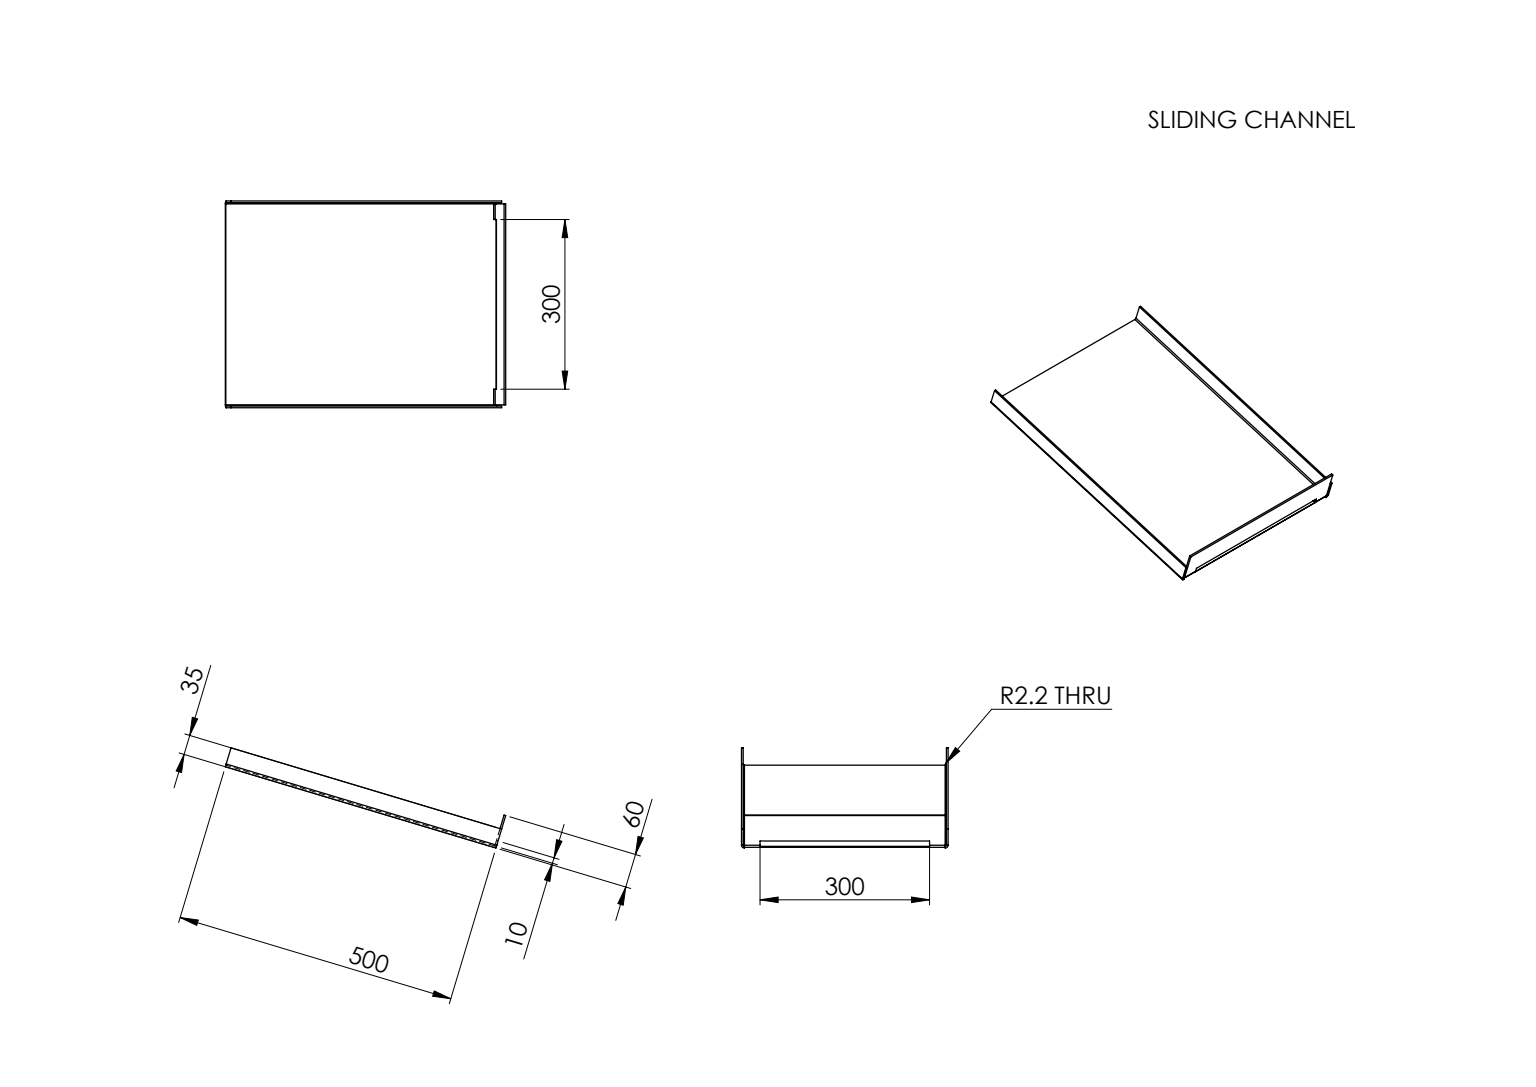
ISO-10303-21;
HEADER;
FILE_DESCRIPTION (('STEP AP214'),
    '1' );
FILE_NAME ('sliding channel.step',
    '2026-10-27T17:01:19',
    ( '' ),
    ( '' ),
    'SwSTEP 2.0',
    'SolidWorks 2026',
    '' );
FILE_SCHEMA (( 'AUTOMOTIVE_DESIGN' ));
ENDSEC;

DATA;
#28=( NAMED_UNIT ( * ) SI_UNIT ( $, .STERADIAN. ) SOLID_ANGLE_UNIT ( ) );
#45=CARTESIAN_POINT ( 'NONE',  ( 702.5260191523640287, 164.1854586329053518, -177.6000000000005059 ) ) ;
#91=ORIENTED_EDGE ( 'NONE', *, *, #14281, .F. ) ;
#93=DIRECTION ( 'NONE',  ( 0.9578262852211525402, -0.2873478855663419429, -0.000000000000000000 ) ) ;
#109=DIRECTION ( 'NONE',  ( 0.000000000000000000, 0.000000000000000000, 1.000000000000000000 ) ) ;
#110=EDGE_LOOP ( 'NONE', ( #11251, #9027, #7663, #8176 ) ) ;
#120=DIRECTION ( 'NONE',  ( -1.673149720584257832E-16, 4.625616335171366110E-15, 1.000000000000000000 ) ) ;
#125=CARTESIAN_POINT ( 'NONE',  ( 716.7018481736364492, 193.3416907550361827, -179.8000000000001535 ) ) ;
#139=LINE ( 'NONE', #7921, #12453 ) ;
#149=DIRECTION ( 'NONE',  ( 0.000000000000000000, 1.000000000000000000, -4.159212477520619976E-15 ) ) ;
#161=CARTESIAN_POINT ( 'NONE',  ( 112.3905262037967248, 374.6350873459896320, 182.7999999999994714 ) ) ;
#166=FACE_OUTER_BOUND ( 'NONE', #2918, .T. ) ;
#167=AXIS2_PLACEMENT_3D ( 'NONE', #3930, #8417, #10718 ) ;
#172=DIRECTION ( 'NONE',  ( 3.340694023494469140E-16, -4.069768234201303760E-15, -1.000000000000000000 ) ) ;
#175=LINE ( 'NONE', #4721, #7503 ) ;
#188=VECTOR ( 'NONE', #2606, 1000.000000000000000 ) ;
#196=ORIENTED_EDGE ( 'NONE', *, *, #8935, .F. ) ;
#199=CARTESIAN_POINT ( 'NONE',  ( 726.1975094929949819, 167.5243180396262801, -149.9999999999986358 ) ) ;
#226=ORIENTED_EDGE ( 'NONE', *, *, #14281, .T. ) ;
#256=VECTOR ( 'NONE', #3741, 1000.000000000000000 ) ;
#288=DIRECTION ( 'NONE',  ( -0.2873478855663281206, -0.9578262852211566480, -1.261617073437843370E-13 ) ) ;
#298=ORIENTED_EDGE ( 'NONE', *, *, #11153, .T. ) ;
#310=CARTESIAN_POINT ( 'NONE',  ( 229.2257385731833779, 308.4724102386176128, -177.6000000000002217 ) ) ;
#334=DIRECTION ( 'NONE',  ( 1.501925087425806625E-16, 4.055197736049677764E-15, 1.000000000000000000 ) ) ;
#367=DIRECTION ( 'NONE',  ( -1.102263794767363534E-15, -3.674212649225433764E-15, -1.000000000000000000 ) ) ;
#376=ORIENTED_EDGE ( 'NONE', *, *, #2427, .F. ) ;
#380=AXIS2_PLACEMENT_3D ( 'NONE', #4209, #11878, #1767 ) ;
#381=DIRECTION ( 'NONE',  ( -0.9578262852211513190, 0.2873478855663454956, -1.110223024625156540E-15 ) ) ;
#394=DIRECTION ( 'NONE',  ( -0.9578262852211506528, 0.2873478855663477161, -0.000000000000000000 ) ) ;
#425=DIRECTION ( 'NONE',  ( -0.9578262852211525402, 0.2873478855663419429, 0.000000000000000000 ) ) ;
#430=EDGE_CURVE ( 'NONE', #7561, #12673, #10485, .T. ) ;
#455=CIRCLE ( 'NONE', #2828, 2.199999999999757705 ) ;
#461=ORIENTED_EDGE ( 'NONE', *, *, #7179, .T. ) ;
#527=CARTESIAN_POINT ( 'NONE',  ( 710.3801946911773939, 172.2695124801716702, -149.9999999999992610 ) ) ;
#547=EDGE_CURVE ( 'NONE', #6337, #5936, #10420, .T. ) ;
#554=DIRECTION ( 'NONE',  ( 0.2873478855663502141, 0.9578262852211498757, -8.036520471939056366E-30 ) ) ;
#567=PLANE ( 'NONE',  #5021 ) ;
#582=CARTESIAN_POINT ( 'NONE',  ( 228.5935732249375292, 306.3651924111313178, -177.6000000000005059 ) ) ;
#597=CARTESIAN_POINT ( 'NONE',  ( 227.7315295682386704, 303.4917135554700280, 177.6000000000001648 ) ) ;
#618=( NAMED_UNIT ( * ) PLANE_ANGLE_UNIT ( ) SI_UNIT ( $, .RADIAN. ) );
#639=ORIENTED_EDGE ( 'NONE', *, *, #9821, .F. ) ;
#647=EDGE_CURVE ( 'NONE', #9997, #6920, #13349, .T. ) ;
#666=EDGE_LOOP ( 'NONE', ( #7423, #9314, #1783, #13496 ) ) ;
#673=CARTESIAN_POINT ( 'NONE',  ( 723.8855453127954434, 217.2873478855664473, 177.5999999999999659 ) ) ;
#683=EDGE_CURVE ( 'NONE', #8002, #5236, #4892, .T. ) ;
#698=EDGE_CURVE ( 'NONE', #10093, #9718, #13285, .T. ) ;
#702=ORIENTED_EDGE ( 'NONE', *, *, #13069, .F. ) ;
#711=EDGE_LOOP ( 'NONE', ( #2678, #10963, #7797, #8249 ) ) ;
#715=VECTOR ( 'NONE', #5972, 1000.000000000000000 ) ;
#733=DIRECTION ( 'NONE',  ( -0.9578262852211513190, 0.2873478855663453846, -1.110223024625157329E-15 ) ) ;
#754=ORIENTED_EDGE ( 'NONE', *, *, #8240, .F. ) ;
#764=EDGE_CURVE ( 'NONE', #11071, #8976, #2432, .T. ) ;
#769=EDGE_CURVE ( 'NONE', #10293, #10481, #1167, .T. ) ;
#777=EDGE_LOOP ( 'NONE', ( #999, #2194, #1865, #13253 ) ) ;
#794=CARTESIAN_POINT ( 'NONE',  ( 237.7887055630607733, 337.0156335382104089, 182.7999999999996135 ) ) ;
#795=CARTESIAN_POINT ( 'NONE',  ( 229.2257385731836621, 308.4724102386199434, 182.7999999999996135 ) ) ;
#826=ORIENTED_EDGE ( 'NONE', *, *, #3158, .T. ) ;
#831=ORIENTED_EDGE ( 'NONE', *, *, #4383, .F. ) ;
#834=DIRECTION ( 'NONE',  ( -0.9578262852211507639, 0.2873478855663477716, 0.000000000000000000 ) ) ;
#837=ORIENTED_EDGE ( 'NONE', *, *, #10575, .F. ) ;
#880=EDGE_CURVE ( 'NONE', #1859, #4991, #1474, .T. ) ;
#884=ORIENTED_EDGE ( 'NONE', *, *, #11917, .F. ) ;
#897=AXIS2_PLACEMENT_3D ( 'NONE', #6006, #10504, #7188 ) ;
#898=VECTOR ( 'NONE', #9160, 1000.000000000000114 ) ;
#899=LINE ( 'NONE', #11699, #906 ) ;
#906=VECTOR ( 'NONE', #6251, 1000.000000000000227 ) ;
#944=AXIS2_PLACEMENT_3D ( 'NONE', #11376, #3638, #8117 ) ;
#971=PLANE ( 'NONE',  #3973 ) ;
#999=ORIENTED_EDGE ( 'NONE', *, *, #2229, .F. ) ;
#1013=ORIENTED_EDGE ( 'NONE', *, *, #8894, .F. ) ;
#1016=FACE_OUTER_BOUND ( 'NONE', #7060, .T. ) ;
#1061=ADVANCED_BREP_SHAPE_REPRESENTATION ( '', ( #7422, #9440 ), #13701 ) ;
#1096=EDGE_LOOP ( 'NONE', ( #2757, #837, #2555, #2386, #1528, #4159 ) ) ;
#1140=DIRECTION ( 'NONE',  ( 0.9578262852211485434, -0.2873478855663546550, 0.000000000000000000 ) ) ;
#1150=AXIS2_PLACEMENT_3D ( 'NONE', #673, #6229, #6519 ) ;
#1157=ORIENTED_EDGE ( 'NONE', *, *, #5120, .F. ) ;
#1167=LINE ( 'NONE', #4581, #5578 ) ;
#1172=ORIENTED_EDGE ( 'NONE', *, *, #4383, .T. ) ;
#1174=VECTOR ( 'NONE', #12504, 1000.000000000000114 ) ;
#1197=DIRECTION ( 'NONE',  ( 0.000000000000000000, 0.000000000000000000, 1.000000000000000000 ) ) ;
#1217=EDGE_LOOP ( 'NONE', ( #14260, #12001, #10390, #9108 ) ) ;
#1237=DIRECTION ( 'NONE',  ( 0.9578262852211507639, -0.2873478855663477716, 0.000000000000000000 ) ) ;
#1239=DIRECTION ( 'NONE',  ( -3.340694023494469140E-16, 4.069768234201303760E-15, 1.000000000000000000 ) ) ;
#1255=ORIENTED_EDGE ( 'NONE', *, *, #4794, .T. ) ;
#1292=ORIENTED_EDGE ( 'NONE', *, *, #7379, .F. ) ;
#1303=( LENGTH_UNIT ( ) NAMED_UNIT ( * ) SI_UNIT ( .MILLI., .METRE. ) );
#1316=DIRECTION ( 'NONE',  ( 9.304756960132325412E-16, 6.965275210156238168E-15, 1.000000000000000000 ) ) ;
#1329=DIRECTION ( 'NONE',  ( 0.000000000000000000, -1.000000000000000000, 4.625616335171366110E-15 ) ) ;
#1331=FACE_OUTER_BOUND ( 'NONE', #711, .T. ) ;
#1355=ORIENTED_EDGE ( 'NONE', *, *, #8452, .F. ) ;
#1370=( NAMED_UNIT ( * ) PLANE_ANGLE_UNIT ( ) SI_UNIT ( $, .RADIAN. ) );
#1452=DIRECTION ( 'NONE',  ( -0.2873478855663461062, -0.9578262852211510969, 0.000000000000000000 ) ) ;
#1454=CARTESIAN_POINT ( 'NONE',  ( 229.2257385731836621, 308.4724102386185223, -182.8000000000004945 ) ) ;
#1457=EDGE_CURVE ( 'NONE', #9718, #6337, #5337, .T. ) ;
#1462=ADVANCED_FACE ( 'NONE', ( #13237 ), #971, .F. ) ;
#1470=CARTESIAN_POINT ( 'NONE',  ( 706.6446721788142895, 159.8177707722969672, 177.6000000000001933 ) ) ;
#1474=LINE ( 'NONE', #3622, #8347 ) ;
#1475=EDGE_LOOP ( 'NONE', ( #7036, #7021, #298, #13292 ) ) ;
#1479=ORIENTED_EDGE ( 'NONE', *, *, #764, .F. ) ;
#1482=ORIENTED_EDGE ( 'NONE', *, *, #8935, .T. ) ;
#1515=EDGE_CURVE ( 'NONE', #12673, #2108, #9837, .T. ) ;
#1525=EDGE_CURVE ( 'NONE', #2008, #2622, #11004, .T. ) ;
#1528=ORIENTED_EDGE ( 'NONE', *, *, #4356, .F. ) ;
#1535=CARTESIAN_POINT ( 'NONE',  ( 726.1975094929949819, 167.5243180396262801, -149.9999999999986358 ) ) ;
#1558=DIRECTION ( 'NONE',  ( 0.000000000000000000, 0.000000000000000000, 1.000000000000000000 ) ) ;
#1577=EDGE_CURVE ( 'NONE', #12373, #10093, #9834, .T. ) ;
#1582=EDGE_CURVE ( 'NONE', #14148, #11328, #2371, .T. ) ;
#1598=ADVANCED_FACE ( 'NONE', ( #13528 ), #2447, .F. ) ;
#1607=ORIENTED_EDGE ( 'NONE', *, *, #3104, .F. ) ;
#1608=LINE ( 'NONE', #6260, #8458 ) ;
#1614=AXIS2_PLACEMENT_3D ( 'NONE', #5274, #13367, #12115 ) ;
#1640=VECTOR ( 'NONE', #9507, 1000.000000000000114 ) ;
#1652=VERTEX_POINT ( 'NONE', #3566 ) ;
#1654=ORIENTED_EDGE ( 'NONE', *, *, #6129, .F. ) ;
#1661=CARTESIAN_POINT ( 'NONE',  ( 604.3113219698392413, -181.2933965909535914, -182.7999999999974250 ) ) ;
#1680=DIRECTION ( 'NONE',  ( -1.000000000000000000, 5.337610695313498298E-15, 0.000000000000000000 ) ) ;
#1687=ADVANCED_FACE ( 'NONE', ( #6948 ), #5621, .T. ) ;
#1725=DIRECTION ( 'NONE',  ( -0.2873478855663455511, -0.9578262852211514300, 4.074758502541097232E-16 ) ) ;
#1744=CARTESIAN_POINT ( 'NONE',  ( 706.6446721788141758, 159.8177707722969956, 177.6000000000005627 ) ) ;
#1766=UNCERTAINTY_MEASURE_WITH_UNIT (LENGTH_MEASURE( 1.000000000000000082E-05 ), #1303, 'distance_accuracy_value', 'NONE');
#1767=DIRECTION ( 'NONE',  ( -1.000000000000000000, 0.000000000000000000, 0.000000000000000000 ) ) ;
#1783=ORIENTED_EDGE ( 'NONE', *, *, #10703, .F. ) ;
#1811=VECTOR ( 'NONE', #8380, 1000.000000000000227 ) ;
#1821=EDGE_CURVE ( 'NONE', #12673, #7913, #13600, .T. ) ;
#1844=CARTESIAN_POINT ( 'NONE',  ( 604.3113219698374223, -181.2933965909537903, 177.6000000000015575 ) ) ;
#1851=CIRCLE ( 'NONE', #7037, 5.199999999999760369 ) ;
#1859=VERTEX_POINT ( 'NONE', #1923 ) ;
#1860=AXIS2_PLACEMENT_3D ( 'NONE', #10254, #5816, #9141 ) ;
#1862=CARTESIAN_POINT ( 'NONE',  ( 721.0120664571321640, 218.1493915422654766, 177.5999999999999659 ) ) ;
#1865=ORIENTED_EDGE ( 'NONE', *, *, #6557, .T. ) ;
#1883=PLANE ( 'NONE',  #4671 ) ;
#1891=DIRECTION ( 'NONE',  ( -0.9578262852211513190, 0.2873478855663453846, 0.000000000000000000 ) ) ;
#1923=CARTESIAN_POINT ( 'NONE',  ( 716.7018481736365629, 193.3416907550376322, 182.8000000000001535 ) ) ;
#1951=VECTOR ( 'NONE', #3608, 1000.000000000000227 ) ;
#1955=EDGE_LOOP ( 'NONE', ( #9013, #4556, #6062, #1255 ) ) ;
#1957=CARTESIAN_POINT ( 'NONE',  ( 702.5260191523640287, 164.1854586329053518, -177.6000000000005059 ) ) ;
#1995=VERTEX_POINT ( 'NONE', #6715 ) ;
#2008=VERTEX_POINT ( 'NONE', #4585 ) ;
#2029=DIRECTION ( 'NONE',  ( 0.9578262852211513190, -0.2873478855663453846, 1.110223024625157329E-15 ) ) ;
#2031=ORIENTED_EDGE ( 'NONE', *, *, #1457, .T. ) ;
#2082=ORIENTED_EDGE ( 'NONE', *, *, #12974, .F. ) ;
#2097=AXIS2_PLACEMENT_3D ( 'NONE', #9208, #1237, #3527 ) ;
#2108=VERTEX_POINT ( 'NONE', #6933 ) ;
#2137=ORIENTED_EDGE ( 'NONE', *, *, #7550, .F. ) ;
#2190=DIRECTION ( 'NONE',  ( 0.2873478855663497700, 0.9578262852211499867, 5.078292077360263497E-30 ) ) ;
#2191=FILL_AREA_STYLE_COLOUR ( '', #11800 ) ;
#2194=ORIENTED_EDGE ( 'NONE', *, *, #12145, .F. ) ;
#2200=CARTESIAN_POINT ( 'NONE',  ( 604.3113219698376497, -181.2933965909545861, -149.9999999999986642 ) ) ;
#2202=DIRECTION ( 'NONE',  ( -1.000000000000000000, 0.000000000000000000, 0.000000000000000000 ) ) ;
#2204=ORIENTED_EDGE ( 'NONE', *, *, #7111, .F. ) ;
#2206=PLANE ( 'NONE',  #6110 ) ;
#2211=CARTESIAN_POINT ( 'NONE',  ( 237.7887055630606028, 337.0156335382089310, -179.8000000000007219 ) ) ;
#2229=EDGE_CURVE ( 'NONE', #10293, #1652, #14305, .T. ) ;
#2253=LINE ( 'NONE', #13712, #1951 ) ;
#2258=CARTESIAN_POINT ( 'NONE',  ( 237.7887055630605460, 337.0156335382089310, -179.8000000000007219 ) ) ;
#2295=DIRECTION ( 'NONE',  ( 1.501925087425806625E-16, 4.055197736049677764E-15, 1.000000000000000000 ) ) ;
#2311=CARTESIAN_POINT ( 'NONE',  ( 703.1581845006096501, 166.2926764603917036, -177.6000000000005059 ) ) ;
#2312=AXIS2_PLACEMENT_3D ( 'NONE', #7015, #12474, #288 ) ;
#2371=LINE ( 'NONE', #11516, #898 ) ;
#2379=CARTESIAN_POINT ( 'NONE',  ( 701.6639754956653405, 161.3119797772417883, -177.6000000000005059 ) ) ;
#2386=ORIENTED_EDGE ( 'NONE', *, *, #7087, .T. ) ;
#2423=CARTESIAN_POINT ( 'NONE',  ( 703.1581845006096501, 166.2926764603917036, 150.0000000000013927 ) ) ;
#2427=EDGE_CURVE ( 'NONE', #7561, #9391, #14094, .T. ) ;
#2430=CARTESIAN_POINT ( 'NONE',  ( -1.716263591756835415E-13, -1.266779246227765552E-12, -179.7999999999981355 ) ) ;
#2432=LINE ( 'NONE', #45, #11930 ) ;
#2447=PLANE ( 'NONE',  #10533 ) ;
#2452=VERTEX_POINT ( 'NONE', #12928 ) ;
#2456=CARTESIAN_POINT ( 'NONE',  ( 228.5935732249376429, 306.3651924111320000, -184.8000000000004945 ) ) ;
#2484=DIRECTION ( 'NONE',  ( 1.000000000000000000, 0.000000000000000000, 0.000000000000000000 ) ) ;
#2485=DIRECTION ( 'NONE',  ( 0.9578262852211524292, -0.2873478855663418874, -0.000000000000000000 ) ) ;
#2490=PLANE ( 'NONE',  #13493 ) ;
#2515=ORIENTED_EDGE ( 'NONE', *, *, #3104, .T. ) ;
#2534=ORIENTED_EDGE ( 'NONE', *, *, #13069, .T. ) ;
#2553=VERTEX_POINT ( 'NONE', #6657 ) ;
#2555=ORIENTED_EDGE ( 'NONE', *, *, #9808, .T. ) ;
#2569=FACE_OUTER_BOUND ( 'NONE', #9843, .T. ) ;
#2585=AXIS2_PLACEMENT_3D ( 'NONE', #2423, #4865, #3453 ) ;
#2599=VECTOR ( 'NONE', #7198, 1000.000000000000114 ) ;
#2602=ORIENTED_EDGE ( 'NONE', *, *, #430, .T. ) ;
#2605=CARTESIAN_POINT ( 'NONE',  ( 723.8855453127955570, 217.2873478855649694, -177.6000000000007901 ) ) ;
#2606=DIRECTION ( 'NONE',  ( -0.9578262852210943645, 0.2873478855665353993, 0.000000000000000000 ) ) ;
#2620=CYLINDRICAL_SURFACE ( 'NONE', #897, 2.199999999999701306 ) ;
#2622=VERTEX_POINT ( 'NONE', #4882 ) ;
#2633=LINE ( 'NONE', #6014, #14313 ) ;
#2678=ORIENTED_EDGE ( 'NONE', *, *, #5120, .T. ) ;
#2681=ADVANCED_FACE ( 'NONE', ( #7519 ), #9671, .F. ) ;
#2724=EDGE_LOOP ( 'NONE', ( #12186, #5469, #2534, #13215 ) ) ;
#2726=DIRECTION ( 'NONE',  ( -0.9578262852211525402, 0.2873478855663419429, 0.000000000000000000 ) ) ;
#2757=ORIENTED_EDGE ( 'NONE', *, *, #1525, .T. ) ;
#2780=DIRECTION ( 'NONE',  ( 0.000000000000000000, 0.000000000000000000, 1.000000000000000000 ) ) ;
#2800=CARTESIAN_POINT ( 'NONE',  ( 229.2257385731834063, 308.4724102386176128, -177.6000000000002217 ) ) ;
#2808=CARTESIAN_POINT ( 'NONE',  ( 707.5067158355133188, 162.6912496279604738, 177.6000000000001648 ) ) ;
#2809=ORIENTED_EDGE ( 'NONE', *, *, #9732, .F. ) ;
#2828=AXIS2_PLACEMENT_3D ( 'NONE', #14234, #4122, #8611 ) ;
#2844=DIRECTION ( 'NONE',  ( 0.9578262852211525402, -0.2873478855663419429, -0.000000000000000000 ) ) ;
#2872=FACE_OUTER_BOUND ( 'NONE', #3651, .T. ) ;
#2914=PLANE ( 'NONE',  #1150 ) ;
#2918=EDGE_LOOP ( 'NONE', ( #3461, #2602, #9198, #5501, #6203, #10799 ) ) ;
#2922=EDGE_CURVE ( 'NONE', #1995, #13316, #175, .T. ) ;
#2942=CARTESIAN_POINT ( 'NONE',  ( 227.7315295682386136, 303.4917135554685501, -184.8000000000004945 ) ) ;
#2950=VERTEX_POINT ( 'NONE', #2258 ) ;
#2957=CARTESIAN_POINT ( 'NONE',  ( 708.1388811837593948, 164.7984674554458309, -179.7999999999999261 ) ) ;
#2961=DIRECTION ( 'NONE',  ( 0.2873478855663434972, 0.9578262852211520961, 0.000000000000000000 ) ) ;
#2963=EDGE_CURVE ( 'NONE', #7913, #9391, #3751, .T. ) ;
#2978=DIRECTION ( 'NONE',  ( 1.102263794768336594E-15, 3.674212649225140308E-15, 1.000000000000000000 ) ) ;
#3023=CYLINDRICAL_SURFACE ( 'NONE', #8224, 5.199999999999732836 ) ;
#3025=DIRECTION ( 'NONE',  ( 0.9578262852211513190, -0.2873478855663455511, 1.110223024625158513E-15 ) ) ;
#3044=ADVANCED_FACE ( 'NONE', ( #7360 ), #4933, .T. ) ;
#3075=DIRECTION ( 'NONE',  ( -1.000000000000000000, 0.000000000000000000, 0.000000000000000000 ) ) ;
#3097=ORIENTED_EDGE ( 'NONE', *, *, #14584, .T. ) ;
#3104=EDGE_CURVE ( 'NONE', #13316, #8002, #899, .T. ) ;
#3117=ORIENTED_EDGE ( 'NONE', *, *, #13879, .T. ) ;
#3149=FACE_OUTER_BOUND ( 'NONE', #6673, .T. ) ;
#3158=EDGE_CURVE ( 'NONE', #8163, #7561, #1851, .T. ) ;
#3164=DIRECTION ( 'NONE',  ( -0.2873478855663454401, -0.9578262852211513190, -4.930380657631323784E-32 ) ) ;
#3169=FACE_OUTER_BOUND ( 'NONE', #4143, .T. ) ;
#3216=DIRECTION ( 'NONE',  ( 0.2873478855663502141, 0.9578262852211498757, -8.036520471939056366E-30 ) ) ;
#3217=EDGE_CURVE ( 'NONE', #8002, #8575, #139, .T. ) ;
#3229=ORIENTED_EDGE ( 'NONE', *, *, #7212, .T. ) ;
#3245=LINE ( 'NONE', #5471, #14359 ) ;
#3266=ORIENTED_EDGE ( 'NONE', *, *, #13723, .F. ) ;
#3275=EDGE_LOOP ( 'NONE', ( #5788, #13853, #13254, #3732, #11465, #10434, #1172, #8641 ) ) ;
#3296=APPLICATION_CONTEXT ( 'automotive_design' ) ;
#3301=DIRECTION ( 'NONE',  ( 0.000000000000000000, 0.000000000000000000, -1.000000000000000000 ) ) ;
#3382=DIRECTION ( 'NONE',  ( -0.9578262852210943645, 0.2873478855665353993, 0.000000000000000000 ) ) ;
#3391=EDGE_CURVE ( 'NONE', #12373, #5236, #12571, .T. ) ;
#3432=ORIENTED_EDGE ( 'NONE', *, *, #2963, .F. ) ;
#3446=LINE ( 'NONE', #13495, #9425 ) ;
#3453=DIRECTION ( 'NONE',  ( 1.000000000000000000, 0.000000000000000000, 0.000000000000000000 ) ) ;
#3461=ORIENTED_EDGE ( 'NONE', *, *, #7550, .T. ) ;
#3474=VECTOR ( 'NONE', #733, 1000.000000000000227 ) ;
#3489=EDGE_CURVE ( 'NONE', #12842, #6920, #4009, .T. ) ;
#3507=ORIENTED_EDGE ( 'NONE', *, *, #4667, .T. ) ;
#3524=( LENGTH_UNIT ( ) NAMED_UNIT ( * ) SI_UNIT ( .MILLI., .METRE. ) );
#3527=DIRECTION ( 'NONE',  ( 0.000000000000000000, 0.000000000000000000, 1.000000000000000000 ) ) ;
#3566=CARTESIAN_POINT ( 'NONE',  ( 229.2257385731837758, 308.4724102386206255, 182.7999999999996135 ) ) ;
#3584=DIRECTION ( 'NONE',  ( 0.000000000000000000, 1.000000000000000000, -3.674212649225433764E-15 ) ) ;
#3608=DIRECTION ( 'NONE',  ( 0.2873478855663497700, 0.9578262852211499867, 5.078292077360263497E-30 ) ) ;
#3620=LINE ( 'NONE', #9070, #9246 ) ;
#3622=CARTESIAN_POINT ( 'NONE',  ( 716.7018481736365629, 193.3416907550376322, 182.8000000000001535 ) ) ;
#3638=DIRECTION ( 'NONE',  ( -0.2873478855663456066, -0.9578262852211514300, 7.452506120068652189E-15 ) ) ;
#3646=EDGE_LOOP ( 'NONE', ( #11392, #4600, #8803, #8779, #10365, #1482 ) ) ;
#3651=EDGE_LOOP ( 'NONE', ( #8860, #11368, #11150, #9833 ) ) ;
#3669=DIRECTION ( 'NONE',  ( 0.9578262852211507639, -0.2873478855663477716, 0.000000000000000000 ) ) ;
#3687=FACE_OUTER_BOUND ( 'NONE', #8533, .T. ) ;
#3696=ORIENTED_EDGE ( 'NONE', *, *, #5732, .T. ) ;
#3704=UNCERTAINTY_MEASURE_WITH_UNIT (LENGTH_MEASURE( 1.000000000000000082E-05 ), #3524, 'distance_accuracy_value', 'NONE');
#3720=EDGE_LOOP ( 'NONE', ( #9824, #9905, #9349, #884 ) ) ;
#3732=ORIENTED_EDGE ( 'NONE', *, *, #10575, .T. ) ;
#3733=EDGE_LOOP ( 'NONE', ( #12839, #7716, #3860, #13532 ) ) ;
#3741=DIRECTION ( 'NONE',  ( 0.9578262852211513190, -0.2873478855663455511, 1.110223024625158513E-15 ) ) ;
#3751=LINE ( 'NONE', #13563, #13168 ) ;
#3754=CARTESIAN_POINT ( 'NONE',  ( 703.1581845006096501, 166.2926764603917036, 150.0000000000013927 ) ) ;
#3762=DIRECTION ( 'NONE',  ( -1.148424442117023040E-15, 3.445273326351216045E-16, 1.000000000000000000 ) ) ;
#3775=LINE ( 'NONE', #199, #14158 ) ;
#3776=VECTOR ( 'NONE', #9804, 1000.000000000000000 ) ;
#3793=AXIS2_PLACEMENT_3D ( 'NONE', #7219, #3762, #9585 ) ;
#3800=AXIS2_PLACEMENT_3D ( 'NONE', #10548, #425, #4817 ) ;
#3820=VECTOR ( 'NONE', #6709, 1000.000000000000227 ) ;
#3825=LINE ( 'NONE', #11761, #256 ) ;
#3826=DIRECTION ( 'NONE',  ( 0.000000000000000000, 0.000000000000000000, 1.000000000000000000 ) ) ;
#3829=ORIENTED_EDGE ( 'NONE', *, *, #3158, .F. ) ;
#3838=DIRECTION ( 'NONE',  ( -0.9578262852211498757, 0.2873478855663503251, -1.198990317802636355E-15 ) ) ;
#3844=ORIENTED_EDGE ( 'NONE', *, *, #647, .F. ) ;
#3860=ORIENTED_EDGE ( 'NONE', *, *, #11979, .F. ) ;
#3865=ADVANCED_FACE ( 'NONE', ( #9592 ), #3023, .T. ) ;
#3868=ORIENTED_EDGE ( 'NONE', *, *, #9803, .F. ) ;
#3930=CARTESIAN_POINT ( 'NONE',  ( 703.1581845006096501, 166.2926764603917036, 177.6000000000001648 ) ) ;
#3954=ORIENTED_EDGE ( 'NONE', *, *, #7804, .F. ) ;
#3966=VECTOR ( 'NONE', #11180, 1000.000000000000000 ) ;
#3967=EDGE_LOOP ( 'NONE', ( #7443, #11520, #6970, #12506 ) ) ;
#3973=AXIS2_PLACEMENT_3D ( 'NONE', #14419, #4311, #8870 ) ;
#3974=ORIENTED_EDGE ( 'NONE', *, *, #6287, .T. ) ;
#3999=STYLED_ITEM('',(#14688),#7422);
#4009=LINE ( 'NONE', #8419, #8472 ) ;
#4016=VECTOR ( 'NONE', #2029, 1000.000000000000227 ) ;
#4017=AXIS2_PLACEMENT_3D ( 'NONE', #4689, #367, #3584 ) ;
#4019=CARTESIAN_POINT ( 'NONE',  ( 707.5067158355135462, 173.1315561368708700, 150.0000000000013642 ) ) ;
#4027=ADVANCED_FACE ( 'NONE', ( #1016 ), #5526, .T. ) ;
#4052=VECTOR ( 'NONE', #4785, 1000.000000000000227 ) ;
#4115=CARTESIAN_POINT ( 'NONE',  ( -1.996809568599176514E-13, 4.067926144610258734E-14, 182.7999999999994714 ) ) ;
#4116=DIRECTION ( 'NONE',  ( -0.9578262852211507639, 0.2873478855663477716, -0.000000000000000000 ) ) ;
#4122=DIRECTION ( 'NONE',  ( -1.148424442117026787E-15, 3.445273326351093279E-16, 1.000000000000000000 ) ) ;
#4131=DIRECTION ( 'NONE',  ( 0.000000000000000000, 0.000000000000000000, 1.000000000000000000 ) ) ;
#4143=EDGE_LOOP ( 'NONE', ( #13847, #13186, #8940, #2515 ) ) ;
#4159=ORIENTED_EDGE ( 'NONE', *, *, #7179, .F. ) ;
#4174=CARTESIAN_POINT ( 'NONE',  ( -1.748605424166683430E-13, -1.289150925701384681E-12, -182.7999999999981355 ) ) ;
#4178=DIRECTION ( 'NONE',  ( -0.000000000000000000, -0.000000000000000000, -1.000000000000000000 ) ) ;
#4185=EDGE_CURVE ( 'NONE', #8873, #11836, #5650, .T. ) ;
#4189=CARTESIAN_POINT ( 'NONE',  ( 710.3801946911771665, 172.2695124801717270, 150.0000000000013358 ) ) ;
#4204=EDGE_CURVE ( 'NONE', #2553, #2452, #4727, .T. ) ;
#4209=CARTESIAN_POINT ( 'NONE',  ( 703.1581845006096501, 166.2926764603917036, -177.6000000000005059 ) ) ;
#4225=CIRCLE ( 'NONE', #4706, 5.199999999999707079 ) ;
#4239=AXIS2_PLACEMENT_3D ( 'NONE', #13555, #93, #5798 ) ;
#4244=DIRECTION ( 'NONE',  ( -0.2873478855662748299, -0.9578262852211725242, -1.261617073437831000E-13 ) ) ;
#4272=DIRECTION ( 'NONE',  ( 0.2873478855663418874, 0.9578262852211524292, 0.000000000000000000 ) ) ;
#4275=DIRECTION ( 'NONE',  ( -0.9578262852211498757, 0.2873478855663503251, -1.198990317802636355E-15 ) ) ;
#4311=DIRECTION ( 'NONE',  ( -0.9578262852211499867, 0.2873478855663502696, -1.489419751501264127E-15 ) ) ;
#4323=VECTOR ( 'NONE', #7274, 1000.000000000000000 ) ;
#4338=ORIENTED_EDGE ( 'NONE', *, *, #4667, .F. ) ;
#4347=CARTESIAN_POINT ( 'NONE',  ( 0.000000000000000000, 0.000000000000000000, 0.000000000000000000 ) ) ;
#4350=FACE_OUTER_BOUND ( 'NONE', #666, .T. ) ;
#4356=EDGE_CURVE ( 'NONE', #8976, #1995, #455, .T. ) ;
#4360=DIRECTION ( 'NONE',  ( -0.000000000000000000, -0.000000000000000000, -1.000000000000000000 ) ) ;
#4376=DIRECTION ( 'NONE',  ( -0.9578262852211506528, 0.2873478855663477161, -0.000000000000000000 ) ) ;
#4383=EDGE_CURVE ( 'NONE', #8575, #9997, #6622, .T. ) ;
#4405=ORIENTED_EDGE ( 'NONE', *, *, #6481, .F. ) ;
#4428=DIRECTION ( 'NONE',  ( -1.000000000000000000, 0.000000000000000000, -1.148424442117026787E-15 ) ) ;
#4441=VECTOR ( 'NONE', #8806, 1000.000000000000000 ) ;
#4448=EDGE_CURVE ( 'NONE', #6337, #14518, #9795, .T. ) ;
#4479=CARTESIAN_POINT ( 'NONE',  ( 703.1581845006096501, 166.2926764603917036, -177.6000000000005059 ) ) ;
#4491=ORIENTED_EDGE ( 'NONE', *, *, #430, .F. ) ;
#4493=AXIS2_PLACEMENT_3D ( 'NONE', #9082, #120, #1329 ) ;
#4500=VECTOR ( 'NONE', #2295, 1000.000000000000000 ) ;
#4540=DIRECTION ( 'NONE',  ( 0.2873478855663502141, 0.9578262852211498757, -4.382459307730876264E-15 ) ) ;
#4556=ORIENTED_EDGE ( 'NONE', *, *, #547, .T. ) ;
#4581=CARTESIAN_POINT ( 'NONE',  ( 229.2257385731836621, 308.4724102386199434, 179.7999999999995850 ) ) ;
#4585=CARTESIAN_POINT ( 'NONE',  ( 707.0389973793288618, 162.8315651648156575, -149.9999999999986642 ) ) ;
#4600=ORIENTED_EDGE ( 'NONE', *, *, #13694, .F. ) ;
#4653=EDGE_LOOP ( 'NONE', ( #3954, #5802, #11817, #1355 ) ) ;
#4656=ORIENTED_EDGE ( 'NONE', *, *, #11917, .T. ) ;
#4667=EDGE_CURVE ( 'NONE', #1859, #4684, #10295, .T. ) ;
#4671=AXIS2_PLACEMENT_3D ( 'NONE', #11397, #12578, #149 ) ;
#4684=VERTEX_POINT ( 'NONE', #9714 ) ;
#4689=CARTESIAN_POINT ( 'NONE',  ( 702.5260191523640287, 164.1854586329053518, 177.6000000000001648 ) ) ;
#4706=AXIS2_PLACEMENT_3D ( 'NONE', #5259, #13076, #2961 ) ;
#4721=CARTESIAN_POINT ( 'NONE',  ( 705.2654023280961155, 165.6605111121464518, 177.6000000000000512 ) ) ;
#4727=CIRCLE ( 'NONE', #4961, 2.199999999999757705 ) ;
#4737=ORIENTED_EDGE ( 'NONE', *, *, #12037, .T. ) ;
#4738=VECTOR ( 'NONE', #12771, 1000.000000000000000 ) ;
#4746=AXIS2_PLACEMENT_3D ( 'NONE', #9554, #1725, #11964 ) ;
#4751=AXIS2_PLACEMENT_3D ( 'NONE', #12075, #11994, #1891 ) ;
#4766=AXIS2_PLACEMENT_3D ( 'NONE', #11919, #5085, #6112 ) ;
#4779=LINE ( 'NONE', #9109, #1174 ) ;
#4785=DIRECTION ( 'NONE',  ( -0.2873478855663502141, -0.9578262852211498757, 3.895519384649669193E-15 ) ) ;
#4794=EDGE_CURVE ( 'NONE', #9268, #14518, #9496, .T. ) ;
#4817=DIRECTION ( 'NONE',  ( -0.2873478855663434972, -0.9578262852211520961, 0.000000000000000000 ) ) ;
#4858=CARTESIAN_POINT ( 'NONE',  ( 237.7887055630605744, 337.0156335382089310, -182.8000000000007219 ) ) ;
#4865=DIRECTION ( 'NONE',  ( 1.148424442117023040E-15, -3.445273326351216045E-16, -1.000000000000000000 ) ) ;
#4879=DIRECTION ( 'NONE',  ( -0.2873478855663477161, -0.9578262852211506528, 1.261617073437870380E-13 ) ) ;
#4882=CARTESIAN_POINT ( 'NONE',  ( 708.1388811837596222, 164.7984674554459446, -149.9999999999986642 ) ) ;
#4892=CIRCLE ( 'NONE', #380, 5.199999999999760369 ) ;
#4924=CARTESIAN_POINT ( 'NONE',  ( 708.1388811837591675, 164.7984674554467119, 177.5999999999999091 ) ) ;
#4933=PLANE ( 'NONE',  #12944 ) ;
#4958=EDGE_CURVE ( 'NONE', #12373, #14148, #13252, .T. ) ;
#4961=AXIS2_PLACEMENT_3D ( 'NONE', #3754, #5746, #2484 ) ;
#4991=VERTEX_POINT ( 'NONE', #7230 ) ;
#5021=AXIS2_PLACEMENT_3D ( 'NONE', #1535, #13947, #10619 ) ;
#5034=EDGE_CURVE ( 'NONE', #5667, #2108, #8336, .T. ) ;
#5041=AXIS2_PLACEMENT_3D ( 'NONE', #6315, #4116, #6397 ) ;
#5060=PLANE ( 'NONE',  #4746 ) ;
#5085=DIRECTION ( 'NONE',  ( 0.9578262852211514300, -0.2873478855663454956, 1.110223024625157329E-15 ) ) ;
#5120=EDGE_CURVE ( 'NONE', #2950, #10050, #13071, .T. ) ;
#5159=ORIENTED_EDGE ( 'NONE', *, *, #5304, .F. ) ;
#5162=DIRECTION ( 'NONE',  ( -1.063400795443705011E-15, 3.190202386331112862E-16, 1.000000000000000000 ) ) ;
#5165=EDGE_LOOP ( 'NONE', ( #10161, #226, #13580, #7884 ) ) ;
#5197=FACE_OUTER_BOUND ( 'NONE', #5165, .T. ) ;
#5216=DIRECTION ( 'NONE',  ( 1.078061080328271067E-15, 7.457226491206363694E-15, 1.000000000000000000 ) ) ;
#5236=VERTEX_POINT ( 'NONE', #12378 ) ;
#5238=CARTESIAN_POINT ( 'NONE',  ( 702.5260191523640287, 164.1854586329053518, -177.6000000000005059 ) ) ;
#5244=ORIENTED_EDGE ( 'NONE', *, *, #2922, .F. ) ;
#5259=CARTESIAN_POINT ( 'NONE',  ( 708.1388811837590538, 164.7984674554467404, 177.5999999999999091 ) ) ;
#5274=CARTESIAN_POINT ( 'NONE',  ( 703.1581845006096501, 166.2926764603917036, -149.9999999999986642 ) ) ;
#5288=APPLICATION_CONTEXT ( 'automotive_design' ) ;
#5290=SHAPE_REPRESENTATION ( 'sliding channel', ( #9440 ), #13701 ) ;
#5304=EDGE_CURVE ( 'NONE', #10698, #6810, #8030, .T. ) ;
#5337=LINE ( 'NONE', #14271, #4441 ) ;
#5352=DIRECTION ( 'NONE',  ( -0.2873478855663477161, -0.9578262852211506528, 0.000000000000000000 ) ) ;
#5374=CARTESIAN_POINT ( 'NONE',  ( 703.1581845006096501, 166.2926764603917036, -177.6000000000005059 ) ) ;
#5392=PRODUCT_CONTEXT ( 'NONE', #5288, 'mechanical' ) ;
#5394=EDGE_CURVE ( 'NONE', #9054, #11328, #13722, .T. ) ;
#5432=LINE ( 'NONE', #6396, #6551 ) ;
#5469=ORIENTED_EDGE ( 'NONE', *, *, #5034, .F. ) ;
#5471=CARTESIAN_POINT ( 'NONE',  ( 228.5935732249375008, 306.3651924111313178, -177.6000000000005059 ) ) ;
#5497=CIRCLE ( 'NONE', #5041, 2.199999999999693312 ) ;
#5501=ORIENTED_EDGE ( 'NONE', *, *, #12145, .T. ) ;
#5502=ADVANCED_FACE ( 'NONE', ( #9515 ), #9733, .F. ) ;
#5526=PLANE ( 'NONE',  #10125 ) ;
#5577=FACE_OUTER_BOUND ( 'NONE', #1217, .T. ) ;
#5578=VECTOR ( 'NONE', #5682, 1000.000000000000000 ) ;
#5581=FACE_OUTER_BOUND ( 'NONE', #3646, .T. ) ;
#5618=VECTOR ( 'NONE', #4376, 1000.000000000000114 ) ;
#5621=PLANE ( 'NONE',  #11704 ) ;
#5642=CARTESIAN_POINT ( 'NONE',  ( 707.0389973793289755, 162.8315651648157427, 177.6000000000001648 ) ) ;
#5648=EDGE_LOOP ( 'NONE', ( #9234, #639, #7110, #3266, #11379 ) ) ;
#5649=ADVANCED_FACE ( 'NONE', ( #5577 ), #9864, .F. ) ;
#5650=CIRCLE ( 'NONE', #2585, 5.199999999999760369 ) ;
#5667=VERTEX_POINT ( 'NONE', #6545 ) ;
#5682=DIRECTION ( 'NONE',  ( 0.9578262852211514300, -0.2873478855663452736, 1.110223024625156540E-15 ) ) ;
#5719=LINE ( 'NONE', #7996, #3966 ) ;
#5732=EDGE_CURVE ( 'NONE', #6920, #7913, #12588, .T. ) ;
#5746=DIRECTION ( 'NONE',  ( 1.148424442117023040E-15, -3.445273326351216045E-16, -1.000000000000000000 ) ) ;
#5753=PLANE ( 'NONE',  #1860 ) ;
#5762=PLANE ( 'NONE',  #4493 ) ;
#5788=ORIENTED_EDGE ( 'NONE', *, *, #9279, .F. ) ;
#5798=DIRECTION ( 'NONE',  ( -0.2873478855663419984, -0.9578262852211524292, -4.803849625782173317E-14 ) ) ;
#5801=( NAMED_UNIT ( * ) SI_UNIT ( $, .STERADIAN. ) SOLID_ANGLE_UNIT ( ) );
#5802=ORIENTED_EDGE ( 'NONE', *, *, #11544, .T. ) ;
#5816=DIRECTION ( 'NONE',  ( 0.9578262852211514300, -0.2873478855663454956, 1.021394162290354552E-15 ) ) ;
#5823=DIRECTION ( 'NONE',  ( 0.2873478855663417764, 0.9578262852211525402, -6.938893903907204712E-15 ) ) ;
#5839=DIRECTION ( 'NONE',  ( 1.416419855379454792E-15, -4.619333907680102023E-16, -1.000000000000000000 ) ) ;
#5858=DIRECTION ( 'NONE',  ( 0.9578262852211504308, -0.2873478855663483267, 0.000000000000000000 ) ) ;
#5884=VECTOR ( 'NONE', #6082, 1000.000000000000227 ) ;
#5890=DIRECTION ( 'NONE',  ( 0.000000000000000000, -1.000000000000000000, 6.965275210156238168E-15 ) ) ;
#5914=EDGE_CURVE ( 'NONE', #10093, #14518, #2633, .T. ) ;
#5931=ADVANCED_FACE ( 'NONE', ( #12880 ), #6238, .F. ) ;
#5936=VERTEX_POINT ( 'NONE', #13925 ) ;
#5963=CARTESIAN_POINT ( 'NONE',  ( 706.6446721788141758, 159.8177707722969956, 177.6000000000005627 ) ) ;
#5972=DIRECTION ( 'NONE',  ( -0.9578262852211513190, 0.2873478855663454956, -1.110223024625156540E-15 ) ) ;
#6006=CARTESIAN_POINT ( 'NONE',  ( 703.1581845006096501, 166.2926764603917036, -177.6000000000005059 ) ) ;
#6014=CARTESIAN_POINT ( 'NONE',  ( 708.1388811837593948, 164.7984674554458593, -182.7999999999998977 ) ) ;
#6020=EDGE_CURVE ( 'NONE', #11328, #8163, #8063, .T. ) ;
#6049=PRODUCT ( 'sliding channel', 'sliding channel', '', ( #5392 ) ) ;
#6061=CIRCLE ( 'NONE', #8414, 5.199999999999715961 ) ;
#6062=ORIENTED_EDGE ( 'NONE', *, *, #10983, .T. ) ;
#6070=VECTOR ( 'NONE', #5162, 1000.000000000000000 ) ;
#6082=DIRECTION ( 'NONE',  ( -0.2873478855663454401, -0.9578262852211513190, -4.930380657631323784E-32 ) ) ;
#6094=DIRECTION ( 'NONE',  ( -0.9578262852211512079, 0.2873478855663461617, -1.110223024625162260E-15 ) ) ;
#6103=LINE ( 'NONE', #5963, #1640 ) ;
#6110=AXIS2_PLACEMENT_3D ( 'NONE', #11213, #9076, #4428 ) ;
#6112=DIRECTION ( 'NONE',  ( 0.2873478855663454401, 0.9578262852211513190, 0.000000000000000000 ) ) ;
#6125=CARTESIAN_POINT ( 'NONE',  ( 723.8855453127956707, 217.2873478855649694, -177.6000000000007617 ) ) ;
#6127=DIRECTION ( 'NONE',  ( -0.9578262852211500977, 0.2873478855663498255, -1.110223024625158907E-15 ) ) ;
#6129=EDGE_CURVE ( 'NONE', #11431, #1652, #6061, .T. ) ;
#6154=STYLED_ITEM ( 'NONE', ( #11475 ), #1061 ) ;
#6180=CARTESIAN_POINT ( 'NONE',  ( 601.4378431141736883, -180.4313529342554432, 150.0000000000013358 ) ) ;
#6203=ORIENTED_EDGE ( 'NONE', *, *, #769, .T. ) ;
#6229=DIRECTION ( 'NONE',  ( -0.2873478855663487708, -0.9578262852211504308, 3.876982066721826743E-15 ) ) ;
#6234=ORIENTED_EDGE ( 'NONE', *, *, #8635, .F. ) ;
#6238=PLANE ( 'NONE',  #10536 ) ;
#6251=DIRECTION ( 'NONE',  ( 0.9578262852211498757, -0.2873478855663502141, 1.489419751501264324E-15 ) ) ;
#6260=CARTESIAN_POINT ( 'NONE',  ( 601.4378431141741430, -180.4313529342555569, -149.9999999999986642 ) ) ;
#6277=ORIENTED_EDGE ( 'NONE', *, *, #4185, .T. ) ;
#6287=EDGE_CURVE ( 'NONE', #13316, #12842, #7135, .T. ) ;
#6300=CARTESIAN_POINT ( 'NONE',  ( 227.7315295682384999, 303.4917135554678680, -177.6000000000009038 ) ) ;
#6315=CARTESIAN_POINT ( 'NONE',  ( 229.2257385731838042, 308.4724102386206255, 177.5999999999999091 ) ) ;
#6335=PLANE ( 'NONE',  #12465 ) ;
#6337=VERTEX_POINT ( 'NONE', #1454 ) ;
#6342=DIRECTION ( 'NONE',  ( 0.000000000000000000, -1.067522139062705339E-14, -1.000000000000000000 ) ) ;
#6386=ADVANCED_FACE ( 'NONE', ( #3149 ), #9642, .F. ) ;
#6396=CARTESIAN_POINT ( 'NONE',  ( 723.3240306373311341, 157.9460551874148564, 150.0000000000013642 ) ) ;
#6397=DIRECTION ( 'NONE',  ( 0.2873478855663431086, 0.9578262852211520961, 1.261617073437853688E-14 ) ) ;
#6400=AXIS2_PLACEMENT_3D ( 'NONE', #4479, #7662, #1140 ) ;
#6404=CARTESIAN_POINT ( 'NONE',  ( 703.1581845006096501, 166.2926764603917036, -177.6000000000005059 ) ) ;
#6417=DIRECTION ( 'NONE',  ( 1.000000000000000000, 0.000000000000000000, 0.000000000000000000 ) ) ;
#6444=ADVANCED_FACE ( 'NONE', ( #11027 ), #9934, .F. ) ;
#6445=CIRCLE ( 'NONE', #6618, 5.199999999999760369 ) ;
#6457=CARTESIAN_POINT ( 'NONE',  ( 707.5067158355136598, 162.6912496279593938, -177.6000000000005059 ) ) ;
#6464=CARTESIAN_POINT ( 'NONE',  ( 707.5067158355135462, 162.6912496279604170, -177.6000000000005059 ) ) ;
#6481=EDGE_CURVE ( 'NONE', #11836, #2452, #5432, .T. ) ;
#6491=DIRECTION ( 'NONE',  ( -0.2873478855663461062, -0.9578262852211510969, 6.938893903907199190E-15 ) ) ;
#6492=ORIENTED_EDGE ( 'NONE', *, *, #7165, .F. ) ;
#6501=ADVANCED_FACE ( 'NONE', ( #11912 ), #1883, .F. ) ;
#6519=DIRECTION ( 'NONE',  ( 0.9578262852211503198, -0.2873478855663487153, 0.000000000000000000 ) ) ;
#6545=CARTESIAN_POINT ( 'NONE',  ( 228.5935732249376429, 306.3651924111320568, -177.6000000000005059 ) ) ;
#6551=VECTOR ( 'NONE', #13259, 1000.000000000000114 ) ;
#6555=LINE ( 'NONE', #8842, #7988 ) ;
#6557=EDGE_CURVE ( 'NONE', #2108, #11431, #5719, .T. ) ;
#6593=DIRECTION ( 'NONE',  ( 0.9578262852211507639, -0.2873478855663477716, 0.000000000000000000 ) ) ;
#6596=ORIENTED_EDGE ( 'NONE', *, *, #5034, .T. ) ;
#6610=VECTOR ( 'NONE', #5823, 1000.000000000000000 ) ;
#6618=AXIS2_PLACEMENT_3D ( 'NONE', #8852, #4360, #2202 ) ;
#6622=LINE ( 'NONE', #13400, #12969 ) ;
#6627=LINE ( 'NONE', #12002, #12047 ) ;
#6628=CYLINDRICAL_SURFACE ( 'NONE', #10117, 2.199999999999730171 ) ;
#6631=ORIENTED_EDGE ( 'NONE', *, *, #8894, .T. ) ;
#6644=CARTESIAN_POINT ( 'NONE',  ( 707.5067158355137735, 173.1315561368707847, -149.9999999999986642 ) ) ;
#6652=SHAPE_DEFINITION_REPRESENTATION ( #8658, #5290 ) ;
#6657=CARTESIAN_POINT ( 'NONE',  ( 705.2654023280957745, 165.6605111121449738, 150.0000000000013358 ) ) ;
#6673=EDGE_LOOP ( 'NONE', ( #3868, #4656, #3507, #11748 ) ) ;
#6700=DIRECTION ( 'NONE',  ( -0.9578262852211507639, 0.2873478855663477716, -0.000000000000000000 ) ) ;
#6709=DIRECTION ( 'NONE',  ( -0.2873478855663502141, -0.9578262852211498757, -4.782469237902382669E-30 ) ) ;
#6715=CARTESIAN_POINT ( 'NONE',  ( 705.2654023280962292, 165.6605111121449738, -149.9999999999986642 ) ) ;
#6760=CARTESIAN_POINT ( 'NONE',  ( 229.2257385731837473, 308.4724102386206255, 177.5999999999999091 ) ) ;
#6768=CARTESIAN_POINT ( 'NONE',  ( 103.1953938656736227, 343.9846462189121326, -1.410137047767614819E-12 ) ) ;
#6773=VECTOR ( 'NONE', #7307, 1000.000000000000114 ) ;
#6810=VERTEX_POINT ( 'NONE', #4019 ) ;
#6817=VECTOR ( 'NONE', #3382, 1000.000000000000000 ) ;
#6822=ADVANCED_FACE ( 'NONE', ( #12045 ), #2914, .F. ) ;
#6848=DIRECTION ( 'NONE',  ( 0.9578262852211498757, -0.2873478855663502141, 1.489419751501263930E-15 ) ) ;
#6912=CARTESIAN_POINT ( 'NONE',  ( 229.2257385731834063, 308.4724102386176128, -177.6000000000002217 ) ) ;
#6920=VERTEX_POINT ( 'NONE', #1862 ) ;
#6933=CARTESIAN_POINT ( 'NONE',  ( 228.5935732249376997, 306.3651924111334779, 177.6000000000001648 ) ) ;
#6948=FACE_OUTER_BOUND ( 'NONE', #777, .T. ) ;
#6956=LINE ( 'NONE', #11451, #13205 ) ;
#6970=ORIENTED_EDGE ( 'NONE', *, *, #7165, .T. ) ;
#6984=DIRECTION ( 'NONE',  ( 3.340694023494469140E-16, -4.069768234201303760E-15, -1.000000000000000000 ) ) ;
#7014=ADVANCED_FACE ( 'NONE', ( #11495 ), #5753, .F. ) ;
#7015=CARTESIAN_POINT ( 'NONE',  ( 708.1388811837593948, 164.7984674554466835, -177.6000000000002217 ) ) ;
#7021=ORIENTED_EDGE ( 'NONE', *, *, #4794, .F. ) ;
#7036=ORIENTED_EDGE ( 'NONE', *, *, #5914, .T. ) ;
#7037=AXIS2_PLACEMENT_3D ( 'NONE', #14015, #2780, #1680 ) ;
#7060=EDGE_LOOP ( 'NONE', ( #6596, #13558, #10966, #4405, #6631, #461, #1479, #11941 ) ) ;
#7087=EDGE_CURVE ( 'NONE', #10436, #1995, #1608, .T. ) ;
#7093=( GEOMETRIC_REPRESENTATION_CONTEXT ( 3 ) GLOBAL_UNCERTAINTY_ASSIGNED_CONTEXT ( ( #1766 ) ) GLOBAL_UNIT_ASSIGNED_CONTEXT ( ( #1303, #13492, #28 ) ) REPRESENTATION_CONTEXT ( 'NONE', 'WORKASPACE' ) );
#7107=ADVANCED_FACE ( 'NONE', ( #3169 ), #6335, .F. ) ;
#7108=ADVANCED_FACE ( 'NONE', ( #4350 ), #9743, .T. ) ;
#7110=ORIENTED_EDGE ( 'NONE', *, *, #4448, .T. ) ;
#7111=EDGE_CURVE ( 'NONE', #10050, #10093, #6555, .T. ) ;
#7123=LINE ( 'NONE', #9491, #5884 ) ;
#7126=DIRECTION ( 'NONE',  ( -0.000000000000000000, -0.000000000000000000, -1.000000000000000000 ) ) ;
#7135=LINE ( 'NONE', #10743, #1811 ) ;
#7141=EDGE_LOOP ( 'NONE', ( #10421, #7960, #9453, #1654, #1292 ) ) ;
#7162=DIRECTION ( 'NONE',  ( -0.9578262852211498757, 0.2873478855663503251, -1.198990317802636355E-15 ) ) ;
#7165=EDGE_CURVE ( 'NONE', #4684, #12841, #10920, .T. ) ;
#7167=CARTESIAN_POINT ( 'NONE',  ( 708.1388811837593948, 164.7984674554466835, -179.7999999999999545 ) ) ;
#7179=EDGE_CURVE ( 'NONE', #2008, #8976, #9873, .T. ) ;
#7188=DIRECTION ( 'NONE',  ( 0.9578262852211485434, -0.2873478855663546550, 0.000000000000000000 ) ) ;
#7198=DIRECTION ( 'NONE',  ( -0.2873478855663461062, -0.9578262852211510969, 6.938893903907199190E-15 ) ) ;
#7212=EDGE_CURVE ( 'NONE', #7913, #2553, #3446, .T. ) ;
#7219=CARTESIAN_POINT ( 'NONE',  ( 726.1975094929946408, 167.5243180396263938, 150.0000000000013642 ) ) ;
#7230=CARTESIAN_POINT ( 'NONE',  ( 716.7018481736365629, 193.3416907550376322, 179.8000000000001535 ) ) ;
#7239=VECTOR ( 'NONE', #10856, 1000.000000000000227 ) ;
#7264=ADVANCED_FACE ( 'NONE', ( #12525 ), #9125, .T. ) ;
#7272=AXIS2_PLACEMENT_3D ( 'NONE', #7382, #6127, #11796 ) ;
#7274=DIRECTION ( 'NONE',  ( 1.078061080328271264E-15, 7.457226491206363694E-15, 1.000000000000000000 ) ) ;
#7304=AXIS2_PLACEMENT_3D ( 'NONE', #9502, #6094, #1452 ) ;
#7307=DIRECTION ( 'NONE',  ( -0.9578262852211506528, 0.2873478855663477161, -0.000000000000000000 ) ) ;
#7318=DIRECTION ( 'NONE',  ( -0.9578262852211503198, 0.2873478855663487153, -1.489419751501257816E-15 ) ) ;
#7341=DIRECTION ( 'NONE',  ( -0.2873478855663361697, -0.9578262852211543166, 0.000000000000000000 ) ) ;
#7358=ORIENTED_EDGE ( 'NONE', *, *, #8452, .T. ) ;
#7360=FACE_OUTER_BOUND ( 'NONE', #9559, .T. ) ;
#7375=DIRECTION ( 'NONE',  ( -0.2873478855663502141, -0.9578262852211498757, -4.782469237902382669E-30 ) ) ;
#7379=EDGE_CURVE ( 'NONE', #8163, #11431, #11767, .T. ) ;
#7382=CARTESIAN_POINT ( 'NONE',  ( 716.7018481736364492, 193.3416907550376322, 182.8000000000001535 ) ) ;
#7406=EDGE_CURVE ( 'NONE', #10624, #8163, #6103, .T. ) ;
#7422=MANIFOLD_SOLID_BREP ( 'Cut-Extrude1', #9280 ) ;
#7423=ORIENTED_EDGE ( 'NONE', *, *, #11721, .F. ) ;
#7443=ORIENTED_EDGE ( 'NONE', *, *, #2229, .T. ) ;
#7503=VECTOR ( 'NONE', #6984, 1000.000000000000000 ) ;
#7512=DIRECTION ( 'NONE',  ( 1.000000000000000000, 0.000000000000000000, -0.000000000000000000 ) ) ;
#7519=FACE_OUTER_BOUND ( 'NONE', #3720, .T. ) ;
#7550=EDGE_CURVE ( 'NONE', #14303, #7561, #4779, .T. ) ;
#7552=VECTOR ( 'NONE', #381, 1000.000000000000000 ) ;
#7561=VERTEX_POINT ( 'NONE', #5642 ) ;
#7574=VECTOR ( 'NONE', #3216, 1000.000000000000227 ) ;
#7595=VECTOR ( 'NONE', #5216, 1000.000000000000000 ) ;
#7604=DIRECTION ( 'NONE',  ( 0.2873478855663454401, 0.9578262852211514300, -3.927332483172771155E-15 ) ) ;
#7607=ADVANCED_FACE ( 'NONE', ( #11249 ), #8001, .T. ) ;
#7633=CARTESIAN_POINT ( 'NONE',  ( 707.5067158355133188, 162.6912496279604738, 177.6000000000001648 ) ) ;
#7659=CARTESIAN_POINT ( 'NONE',  ( 604.3113219698371950, -181.2933965909544725, 150.0000000000013358 ) ) ;
#7662=DIRECTION ( 'NONE',  ( -0.000000000000000000, -0.000000000000000000, -1.000000000000000000 ) ) ;
#7663=ORIENTED_EDGE ( 'NONE', *, *, #11675, .F. ) ;
#7670=EDGE_CURVE ( 'NONE', #4684, #1652, #7123, .T. ) ;
#7716=ORIENTED_EDGE ( 'NONE', *, *, #9732, .T. ) ;
#7731=AXIS2_PLACEMENT_3D ( 'NONE', #4115, #12197, #10960 ) ;
#7732=CARTESIAN_POINT ( 'NONE',  ( 707.0389973793288618, 162.8315651648156290, 150.0000000000013358 ) ) ;
#7794=VECTOR ( 'NONE', #9684, 1000.000000000000227 ) ;
#7797=ORIENTED_EDGE ( 'NONE', *, *, #10983, .F. ) ;
#7804=EDGE_CURVE ( 'NONE', #10481, #14303, #9189, .T. ) ;
#7809=VECTOR ( 'NONE', #2485, 1000.000000000000114 ) ;
#7814=CARTESIAN_POINT ( 'NONE',  ( -1.968420164455561244E-13, 3.855132749030457888E-14, 179.7999999999994714 ) ) ;
#7817=AXIS2_PLACEMENT_3D ( 'NONE', #310, #13918, #7341 ) ;
#7818=EDGE_LOOP ( 'NONE', ( #11540, #754, #13242, #3696 ) ) ;
#7827=FACE_OUTER_BOUND ( 'NONE', #13644, .T. ) ;
#7839=EDGE_LOOP ( 'NONE', ( #3229, #10978, #12988, #14318 ) ) ;
#7884=ORIENTED_EDGE ( 'NONE', *, *, #4958, .F. ) ;
#7913=VERTEX_POINT ( 'NONE', #8872 ) ;
#7921=CARTESIAN_POINT ( 'NONE',  ( 604.3113219698374223, -181.2933965909553535, -177.5999999999989143 ) ) ;
#7957=DIRECTION ( 'NONE',  ( -1.063400795443706786E-15, 3.190202386331118779E-16, 1.000000000000000000 ) ) ;
#7960=ORIENTED_EDGE ( 'NONE', *, *, #12950, .F. ) ;
#7970=LINE ( 'NONE', #2211, #6610 ) ;
#7974=AXIS2_PLACEMENT_3D ( 'NONE', #6457, #2978, #9914 ) ;
#7988=VECTOR ( 'NONE', #6491, 1000.000000000000114 ) ;
#7996=CARTESIAN_POINT ( 'NONE',  ( 228.5935732249378987, 306.3651924111343305, 177.6000000000001648 ) ) ;
#8001=CYLINDRICAL_SURFACE ( 'NONE', #12014, 5.199999999999715961 ) ;
#8002=VERTEX_POINT ( 'NONE', #13593 ) ;
#8030=LINE ( 'NONE', #12534, #8259 ) ;
#8032=MECHANICAL_DESIGN_GEOMETRIC_PRESENTATION_REPRESENTATION('',(#6154),#7093);
#8063=LINE ( 'NONE', #2379, #14084 ) ;
#8085=EDGE_CURVE ( 'NONE', #10698, #9444, #13976, .T. ) ;
#8117=DIRECTION ( 'NONE',  ( 0.9578262852211513190, -0.2873478855663455511, 0.000000000000000000 ) ) ;
#8163=VERTEX_POINT ( 'NONE', #11884 ) ;
#8176=ORIENTED_EDGE ( 'NONE', *, *, #5394, .T. ) ;
#8190=CARTESIAN_POINT ( 'NONE',  ( 703.1581845006096501, 166.2926764603917036, 177.6000000000001648 ) ) ;
#8224=AXIS2_PLACEMENT_3D ( 'NONE', #2800, #2726, #6342 ) ;
#8240=EDGE_CURVE ( 'NONE', #9997, #9391, #11815, .T. ) ;
#8249=ORIENTED_EDGE ( 'NONE', *, *, #11979, .T. ) ;
#8259=VECTOR ( 'NONE', #3838, 1000.000000000000114 ) ;
#8277=EDGE_LOOP ( 'NONE', ( #1607, #3974, #14364, #14558 ) ) ;
#8299=EDGE_LOOP ( 'NONE', ( #4491, #8367, #3432, #9472 ) ) ;
#8336=LINE ( 'NONE', #2456, #4500 ) ;
#8347=VECTOR ( 'NONE', #12610, 1000.000000000000000 ) ;
#8367=ORIENTED_EDGE ( 'NONE', *, *, #2427, .T. ) ;
#8380=DIRECTION ( 'NONE',  ( 0.2873478855663502141, 0.9578262852211498757, -4.382459307730876264E-15 ) ) ;
#8381=LINE ( 'NONE', #4858, #4323 ) ;
#8414=AXIS2_PLACEMENT_3D ( 'NONE', #6760, #6700, #12521 ) ;
#8417=DIRECTION ( 'NONE',  ( 0.000000000000000000, 0.000000000000000000, 1.000000000000000000 ) ) ;
#8419=CARTESIAN_POINT ( 'NONE',  ( 721.0120664571321640, 218.1493915422654482, 177.5999999999999659 ) ) ;
#8423=AXIS2_PLACEMENT_3D ( 'NONE', #4174, #8602, #8672 ) ;
#8444=DIRECTION ( 'NONE',  ( -3.340694023494469140E-16, 4.069768234201303760E-15, 1.000000000000000000 ) ) ;
#8451=ORIENTED_EDGE ( 'NONE', *, *, #6287, .F. ) ;
#8452=EDGE_CURVE ( 'NONE', #14303, #10624, #9528, .T. ) ;
#8453=( LENGTH_UNIT ( ) NAMED_UNIT ( * ) SI_UNIT ( .MILLI., .METRE. ) );
#8458=VECTOR ( 'NONE', #7375, 1000.000000000000227 ) ;
#8472=VECTOR ( 'NONE', #10869, 1000.000000000000000 ) ;
#8494=CARTESIAN_POINT ( 'NONE',  ( 721.0120664571322777, 218.1493915422639702, -177.6000000000007617 ) ) ;
#8529=ORIENTED_EDGE ( 'NONE', *, *, #6481, .T. ) ;
#8533=EDGE_LOOP ( 'NONE', ( #2809, #12857, #2204, #1157 ) ) ;
#8551=LINE ( 'NONE', #2942, #13264 ) ;
#8559=ORIENTED_EDGE ( 'NONE', *, *, #9279, .T. ) ;
#8575=VERTEX_POINT ( 'NONE', #6125 ) ;
#8602=DIRECTION ( 'NONE',  ( 9.304756960132325412E-16, 6.965275210156238168E-15, 1.000000000000000000 ) ) ;
#8611=DIRECTION ( 'NONE',  ( -1.000000000000000000, 3.784851220313450466E-14, 0.000000000000000000 ) ) ;
#8635=EDGE_CURVE ( 'NONE', #8873, #10698, #13397, .T. ) ;
#8641=ORIENTED_EDGE ( 'NONE', *, *, #8240, .T. ) ;
#8658=PRODUCT_DEFINITION_SHAPE ( 'NONE', 'NONE',  #14515 ) ;
#8672=DIRECTION ( 'NONE',  ( 0.000000000000000000, -1.000000000000000000, 6.965275210156238168E-15 ) ) ;
#8698=CIRCLE ( 'NONE', #13415, 2.199999999999757705 ) ;
#8724=ADVANCED_FACE ( 'NONE', ( #10906 ), #10967, .F. ) ;
#8775=LINE ( 'NONE', #10918, #10905 ) ;
#8779=ORIENTED_EDGE ( 'NONE', *, *, #1577, .T. ) ;
#8792=LINE ( 'NONE', #582, #12221 ) ;
#8803=ORIENTED_EDGE ( 'NONE', *, *, #3391, .F. ) ;
#8806=DIRECTION ( 'NONE',  ( 2.985317128751799872E-15, 6.087367539060727577E-15, -1.000000000000000000 ) ) ;
#8815=ORIENTED_EDGE ( 'NONE', *, *, #9821, .T. ) ;
#8822=LINE ( 'NONE', #13174, #7595 ) ;
#8842=CARTESIAN_POINT ( 'NONE',  ( 707.5067158355134325, 162.6912496279593370, -179.7999999999999261 ) ) ;
#8852=CARTESIAN_POINT ( 'NONE',  ( 703.1581845006096501, 166.2926764603917036, -177.6000000000005059 ) ) ;
#8860=ORIENTED_EDGE ( 'NONE', *, *, #5304, .T. ) ;
#8870=DIRECTION ( 'NONE',  ( -0.2873478855663502141, -0.9578262852211498757, 0.000000000000000000 ) ) ;
#8872=CARTESIAN_POINT ( 'NONE',  ( 705.2654023280958882, 165.6605111121457981, 177.6000000000001648 ) ) ;
#8873=VERTEX_POINT ( 'NONE', #10450 ) ;
#8894=EDGE_CURVE ( 'NONE', #11836, #2008, #13835, .T. ) ;
#8906=SURFACE_SIDE_STYLE ('',( #14596 ) ) ;
#8920=CARTESIAN_POINT ( 'NONE',  ( 229.2257385731838326, 308.4724102386206255, 179.7999999999995850 ) ) ;
#8935=EDGE_CURVE ( 'NONE', #9718, #5667, #13470, .T. ) ;
#8940=ORIENTED_EDGE ( 'NONE', *, *, #13201, .F. ) ;
#8976=VERTEX_POINT ( 'NONE', #10587 ) ;
#8992=VECTOR ( 'NONE', #7318, 1000.000000000000227 ) ;
#9000=CARTESIAN_POINT ( 'NONE',  ( 708.1388811837590538, 164.7984674554467404, 179.7999999999995850 ) ) ;
#9013=ORIENTED_EDGE ( 'NONE', *, *, #4448, .F. ) ;
#9027=ORIENTED_EDGE ( 'NONE', *, *, #7379, .T. ) ;
#9054=VERTEX_POINT ( 'NONE', #6300 ) ;
#9070=CARTESIAN_POINT ( 'NONE',  ( 708.1388811837593948, 164.7984674554473088, 179.8000000000001819 ) ) ;
#9076=DIRECTION ( 'NONE',  ( 1.148424442117026787E-15, -3.445273326351093279E-16, -1.000000000000000000 ) ) ;
#9082=CARTESIAN_POINT ( 'NONE',  ( 723.8855453127955570, 217.2873478855649694, -177.6000000000007617 ) ) ;
#9108=ORIENTED_EDGE ( 'NONE', *, *, #13201, .T. ) ;
#9109=CARTESIAN_POINT ( 'NONE',  ( 707.5067158355133188, 162.6912496279604738, 177.6000000000001648 ) ) ;
#9125=CYLINDRICAL_SURFACE ( 'NONE', #2097, 5.199999999999704414 ) ;
#9141=DIRECTION ( 'NONE',  ( 0.2873478855663454401, 0.9578262852211513190, 0.000000000000000000 ) ) ;
#9156=UNCERTAINTY_MEASURE_WITH_UNIT (LENGTH_MEASURE( 1.000000000000000082E-05 ), #8453, 'distance_accuracy_value', 'NONE');
#9160=DIRECTION ( 'NONE',  ( -0.9578262852211524292, 0.2873478855663418874, 0.000000000000000000 ) ) ;
#9189=CIRCLE ( 'NONE', #9672, 2.199999999999685318 ) ;
#9198=ORIENTED_EDGE ( 'NONE', *, *, #1515, .T. ) ;
#9208=CARTESIAN_POINT ( 'NONE',  ( 708.1388811837591675, 164.7984674554467119, 177.5999999999999091 ) ) ;
#9234=ORIENTED_EDGE ( 'NONE', *, *, #5394, .F. ) ;
#9239=ADVANCED_FACE ( 'NONE', ( #11309 ), #10349, .T. ) ;
#9243=ORIENTED_EDGE ( 'NONE', *, *, #4958, .T. ) ;
#9246=VECTOR ( 'NONE', #7957, 1000.000000000000000 ) ;
#9268=VERTEX_POINT ( 'NONE', #10279 ) ;
#9279=EDGE_CURVE ( 'NONE', #8873, #9391, #6956, .T. ) ;
#9280=CLOSED_SHELL ( 'NONE', ( #12383, #12488, #14150, #4027, #8724, #7014, #11718, #5931, #3865, #13585, #1598, #13795, #6444, #11546, #10040, #1687, #13936, #7264, #13727, #5502, #2681, #6386, #7108, #14319, #9239, #7107, #7607, #5649, #9692, #6501, #1462, #3044, #6822, #14592, #13058, #11621 ) ) ;
#9307=EDGE_CURVE ( 'NONE', #8575, #12842, #10566, .T. ) ;
#9314=ORIENTED_EDGE ( 'NONE', *, *, #769, .F. ) ;
#9332=CARTESIAN_POINT ( 'NONE',  ( 707.5067158355136598, 162.6912496279593938, -177.6000000000005059 ) ) ;
#9349=ORIENTED_EDGE ( 'NONE', *, *, #880, .F. ) ;
#9360=ORIENTED_EDGE ( 'NONE', *, *, #7087, .F. ) ;
#9391=VERTEX_POINT ( 'NONE', #11820 ) ;
#9418=ORIENTED_EDGE ( 'NONE', *, *, #7212, .F. ) ;
#9425=VECTOR ( 'NONE', #172, 1000.000000000000000 ) ;
#9440=AXIS2_PLACEMENT_3D ( 'NONE', #4347, #14302, #6417 ) ;
#9444=VERTEX_POINT ( 'NONE', #527 ) ;
#9453=ORIENTED_EDGE ( 'NONE', *, *, #9803, .T. ) ;
#9470=CARTESIAN_POINT ( 'NONE',  ( 710.3801946911771665, 172.2695124801717270, 9.266195726029882063E-13 ) ) ;
#9472=ORIENTED_EDGE ( 'NONE', *, *, #1821, .F. ) ;
#9491=CARTESIAN_POINT ( 'NONE',  ( 125.3981793592638923, -37.61945380777919468, 182.7999999999996135 ) ) ;
#9496=LINE ( 'NONE', #1661, #2599 ) ;
#9502=CARTESIAN_POINT ( 'NONE',  ( 707.5067158355134325, 162.6912496279593086, -182.7999999999999261 ) ) ;
#9507=DIRECTION ( 'NONE',  ( -0.9578262852211506528, 0.2873478855663477161, -0.000000000000000000 ) ) ;
#9515=FACE_OUTER_BOUND ( 'NONE', #3967, .T. ) ;
#9528=LINE ( 'NONE', #10327, #11806 ) ;
#9554=CARTESIAN_POINT ( 'NONE',  ( 237.7887055630607733, 337.0156335382104089, 182.7999999999996135 ) ) ;
#9559=EDGE_LOOP ( 'NONE', ( #9789, #9418, #11791, #11391, #8451, #5244, #9360, #2082 ) ) ;
#9566=CARTESIAN_POINT ( 'NONE',  ( 229.2257385731833779, 308.4724102386176128, -177.6000000000002217 ) ) ;
#9570=FACE_OUTER_BOUND ( 'NONE', #1475, .T. ) ;
#9585=DIRECTION ( 'NONE',  ( 1.000000000000000000, 0.000000000000000000, 1.148424442117023040E-15 ) ) ;
#9592=FACE_OUTER_BOUND ( 'NONE', #5648, .T. ) ;
#9642=PLANE ( 'NONE',  #7731 ) ;
#9643=LINE ( 'NONE', #6180, #13501 ) ;
#9663=LINE ( 'NONE', #10620, #715 ) ;
#9671=PLANE ( 'NONE',  #7272 ) ;
#9672=AXIS2_PLACEMENT_3D ( 'NONE', #12120, #6593, #13164 ) ;
#9684=DIRECTION ( 'NONE',  ( -0.2873478855663502141, -0.9578262852211498757, 3.895519384649669193E-15 ) ) ;
#9692=ADVANCED_FACE ( 'NONE', ( #12464 ), #5762, .F. ) ;
#9714=CARTESIAN_POINT ( 'NONE',  ( 237.7887055630607733, 337.0156335382104658, 182.7999999999996135 ) ) ;
#9718=VERTEX_POINT ( 'NONE', #10113 ) ;
#9732=EDGE_CURVE ( 'NONE', #9718, #2950, #7970, .T. ) ;
#9733=PLANE ( 'NONE',  #4766 ) ;
#9743=PLANE ( 'NONE',  #14366 ) ;
#9789=ORIENTED_EDGE ( 'NONE', *, *, #12037, .F. ) ;
#9795=LINE ( 'NONE', #14516, #4016 ) ;
#9803=EDGE_CURVE ( 'NONE', #12598, #1652, #13878, .T. ) ;
#9804=DIRECTION ( 'NONE',  ( 9.463134714538378657E-16, -7.093113185993356941E-16, -1.000000000000000000 ) ) ;
#9808=EDGE_CURVE ( 'NONE', #9444, #10436, #3775, .T. ) ;
#9821=EDGE_CURVE ( 'NONE', #6337, #9054, #10145, .T. ) ;
#9824=ORIENTED_EDGE ( 'NONE', *, *, #11544, .F. ) ;
#9833=ORIENTED_EDGE ( 'NONE', *, *, #8085, .F. ) ;
#9834=CIRCLE ( 'NONE', #2312, 2.199999999999711520 ) ;
#9837=LINE ( 'NONE', #7633, #5618 ) ;
#9843=EDGE_LOOP ( 'NONE', ( #6277, #8529, #10155, #4737, #5159, #6234 ) ) ;
#9864=CYLINDRICAL_SURFACE ( 'NONE', #6400, 2.199999999999701306 ) ;
#9873=LINE ( 'NONE', #14380, #14375 ) ;
#9905=ORIENTED_EDGE ( 'NONE', *, *, #11721, .T. ) ;
#9914=DIRECTION ( 'NONE',  ( 0.000000000000000000, -1.000000000000000000, 3.674212649225140308E-15 ) ) ;
#9924=VECTOR ( 'NONE', #3025, 1000.000000000000000 ) ;
#9931=CARTESIAN_POINT ( 'NONE',  ( 708.1388811837595085, 164.7984674554473941, 177.6000000000000512 ) ) ;
#9934=PLANE ( 'NONE',  #8423 ) ;
#9955=DIRECTION ( 'NONE',  ( -1.000000000000000000, 0.000000000000000000, -1.063400795443704616E-15 ) ) ;
#9997=VERTEX_POINT ( 'NONE', #10334 ) ;
#10017=CARTESIAN_POINT ( 'NONE',  ( 708.1388811837593948, 164.7984674554466835, -177.6000000000002217 ) ) ;
#10032=LINE ( 'NONE', #10256, #12454 ) ;
#10040=ADVANCED_FACE ( 'NONE', ( #1331 ), #11297, .F. ) ;
#10050=VERTEX_POINT ( 'NONE', #125 ) ;
#10088=FILL_AREA_STYLE ('',( #2191 ) ) ;
#10093=VERTEX_POINT ( 'NONE', #7167 ) ;
#10108=DIRECTION ( 'NONE',  ( 1.416419855379454792E-15, -4.619333907680102023E-16, -1.000000000000000000 ) ) ;
#10113=CARTESIAN_POINT ( 'NONE',  ( 229.2257385731833779, 308.4724102386176128, -179.7999999999999545 ) ) ;
#10117=AXIS2_PLACEMENT_3D ( 'NONE', #6912, #13623, #3301 ) ;
#10122=DIRECTION ( 'NONE',  ( -0.9578262852211507639, 0.2873478855663477716, 0.000000000000000000 ) ) ;
#10125=AXIS2_PLACEMENT_3D ( 'NONE', #6768, #7604, #12306 ) ;
#10145=CIRCLE ( 'NONE', #3800, 5.199999999999707079 ) ;
#10155=ORIENTED_EDGE ( 'NONE', *, *, #4204, .F. ) ;
#10161=ORIENTED_EDGE ( 'NONE', *, *, #3391, .T. ) ;
#10189=FACE_OUTER_BOUND ( 'NONE', #1096, .T. ) ;
#10209=ORIENTED_EDGE ( 'NONE', *, *, #13723, .T. ) ;
#10254=CARTESIAN_POINT ( 'NONE',  ( 228.5935732249376429, 306.3651924111320000, -184.8000000000004945 ) ) ;
#10256=CARTESIAN_POINT ( 'NONE',  ( 707.5067158355137735, 173.1315561368708131, 9.221513133484845664E-13 ) ) ;
#10279=CARTESIAN_POINT ( 'NONE',  ( 716.7018481736364492, 193.3416907550361543, -182.8000000000001535 ) ) ;
#10291=DIRECTION ( 'NONE',  ( -0.000000000000000000, -0.000000000000000000, -1.000000000000000000 ) ) ;
#10293=VERTEX_POINT ( 'NONE', #8920 ) ;
#10295=LINE ( 'NONE', #161, #7552 ) ;
#10327=CARTESIAN_POINT ( 'NONE',  ( 707.5067158355132051, 162.6912496279605307, 177.6000000000001648 ) ) ;
#10334=CARTESIAN_POINT ( 'NONE',  ( 723.8855453127956707, 217.2873478855664757, 177.5999999999999375 ) ) ;
#10349=PLANE ( 'NONE',  #10846 ) ;
#10353=VECTOR ( 'NONE', #394, 1000.000000000000114 ) ;
#10358=PLANE ( 'NONE',  #4017 ) ;
#10365=ORIENTED_EDGE ( 'NONE', *, *, #698, .T. ) ;
#10382=SHAPE_REPRESENTATION_RELATIONSHIP ( 'NONE' , 'NONE' ,  #5290, #1061 ) ;
#10390=ORIENTED_EDGE ( 'NONE', *, *, #2922, .T. ) ;
#10397=ORIENTED_EDGE ( 'NONE', *, *, #3489, .T. ) ;
#10420=LINE ( 'NONE', #12919, #10498 ) ;
#10421=ORIENTED_EDGE ( 'NONE', *, *, #7406, .F. ) ;
#10434=ORIENTED_EDGE ( 'NONE', *, *, #3217, .T. ) ;
#10436=VERTEX_POINT ( 'NONE', #6644 ) ;
#10450=CARTESIAN_POINT ( 'NONE',  ( 708.1388811837592812, 164.7984674554459446, 150.0000000000013358 ) ) ;
#10481=VERTEX_POINT ( 'NONE', #9000 ) ;
#10485=LINE ( 'NONE', #2808, #6773 ) ;
#10498=VECTOR ( 'NONE', #13969, 1000.000000000000000 ) ;
#10504=DIRECTION ( 'NONE',  ( -0.000000000000000000, -0.000000000000000000, -1.000000000000000000 ) ) ;
#10514=DIRECTION ( 'NONE',  ( 2.985317128751861403E-15, 6.087367539060710222E-15, -1.000000000000000000 ) ) ;
#10533=AXIS2_PLACEMENT_3D ( 'NONE', #13666, #13813, #13748 ) ;
#10536=AXIS2_PLACEMENT_3D ( 'NONE', #9566, #2844, #11841 ) ;
#10548=CARTESIAN_POINT ( 'NONE',  ( 229.2257385731833779, 308.4724102386176128, -177.6000000000002217 ) ) ;
#10566=LINE ( 'NONE', #2605, #8992 ) ;
#10574=CARTESIAN_POINT ( 'NONE',  ( 701.6639754956653405, 161.3119797772417883, -177.6000000000005059 ) ) ;
#10575=EDGE_CURVE ( 'NONE', #9444, #2622, #12310, .T. ) ;
#10582=EDGE_LOOP ( 'NONE', ( #10882, #8559, #376, #3829, #11569, #91, #11269, #3117, #14006, #1013 ) ) ;
#10587=CARTESIAN_POINT ( 'NONE',  ( 702.5260191523636877, 164.1854586329052381, -149.9999999999986642 ) ) ;
#10593=CIRCLE ( 'NONE', #4239, 5.199999999999733724 ) ;
#10602=MECHANICAL_DESIGN_GEOMETRIC_PRESENTATION_REPRESENTATION('',(#3999),#12473);
#10619=DIRECTION ( 'NONE',  ( -0.9578262852211498757, 0.2873478855663503251, 0.000000000000000000 ) ) ;
#10620=CARTESIAN_POINT ( 'NONE',  ( 237.7887055630607733, 337.0156335382104089, 179.7999999999995850 ) ) ;
#10624=VERTEX_POINT ( 'NONE', #1470 ) ;
#10632=VECTOR ( 'NONE', #4244, 1000.000000000000114 ) ;
#10651=CARTESIAN_POINT ( 'NONE',  ( 707.5067158355136598, 162.6912496279593938, -177.6000000000005059 ) ) ;
#10686=DIRECTION ( 'NONE',  ( -0.9578262852211499867, 0.2873478855663502696, -1.489419751501264127E-15 ) ) ;
#10698=VERTEX_POINT ( 'NONE', #4189 ) ;
#10703=EDGE_CURVE ( 'NONE', #12841, #10293, #6627, .T. ) ;
#10718=DIRECTION ( 'NONE',  ( -1.000000000000000000, 0.000000000000000000, 0.000000000000000000 ) ) ;
#10721=CARTESIAN_POINT ( 'NONE',  ( 705.2654023280958882, 165.6605111121457981, -177.6000000000005059 ) ) ;
#10727=CARTESIAN_POINT ( 'NONE',  ( 707.5067158355135462, 162.6912496279608717, 177.6000000000001648 ) ) ;
#10743=CARTESIAN_POINT ( 'NONE',  ( 721.0120664571322777, 218.1493915422639986, -177.6000000000007617 ) ) ;
#10775=DIRECTION ( 'NONE',  ( 0.9578262852211524292, -0.2873478855663418874, -0.000000000000000000 ) ) ;
#10799=ORIENTED_EDGE ( 'NONE', *, *, #7804, .T. ) ;
#10833=LINE ( 'NONE', #5238, #10841 ) ;
#10841=VECTOR ( 'NONE', #14239, 1000.000000000000000 ) ;
#10846=AXIS2_PLACEMENT_3D ( 'NONE', #13596, #1197, #11168 ) ;
#10850=CARTESIAN_POINT ( 'NONE',  ( 716.7018481736364492, 193.3416907550361827, -179.8000000000001535 ) ) ;
#10856=DIRECTION ( 'NONE',  ( -0.9578262852211503198, 0.2873478855663487153, -1.489419751501258013E-15 ) ) ;
#10869=DIRECTION ( 'NONE',  ( -3.125627884642896034E-16, 4.141456947151826978E-15, 1.000000000000000000 ) ) ;
#10882=ORIENTED_EDGE ( 'NONE', *, *, #4185, .F. ) ;
#10895=PLANE ( 'NONE',  #11773 ) ;
#10905=VECTOR ( 'NONE', #2190, 1000.000000000000227 ) ;
#10906=FACE_OUTER_BOUND ( 'NONE', #110, .T. ) ;
#10918=CARTESIAN_POINT ( 'NONE',  ( 716.7018481736364492, 193.3416907550376322, 179.8000000000001535 ) ) ;
#10920=LINE ( 'NONE', #794, #3776 ) ;
#10959=CARTESIAN_POINT ( 'NONE',  ( 708.1388811837590538, 164.7984674554467404, 177.5999999999999091 ) ) ;
#10960=DIRECTION ( 'NONE',  ( -1.000000000000000000, 0.000000000000000000, -1.063400795443704616E-15 ) ) ;
#10963=ORIENTED_EDGE ( 'NONE', *, *, #11153, .F. ) ;
#10966=ORIENTED_EDGE ( 'NONE', *, *, #13526, .F. ) ;
#10967=PLANE ( 'NONE',  #4751 ) ;
#10978=ORIENTED_EDGE ( 'NONE', *, *, #4204, .T. ) ;
#10983=EDGE_CURVE ( 'NONE', #5936, #9268, #3825, .T. ) ;
#11004=CIRCLE ( 'NONE', #1614, 5.199999999999760369 ) ;
#11027=FACE_OUTER_BOUND ( 'NONE', #1955, .T. ) ;
#11071=VERTEX_POINT ( 'NONE', #1957 ) ;
#11120=DIRECTION ( 'NONE',  ( -3.125627884642896034E-16, 4.141456947151826978E-15, 1.000000000000000000 ) ) ;
#11126=LINE ( 'NONE', #14591, #6817 ) ;
#11150=ORIENTED_EDGE ( 'NONE', *, *, #9808, .F. ) ;
#11153=EDGE_CURVE ( 'NONE', #9268, #10050, #8822, .T. ) ;
#11161=EDGE_LOOP ( 'NONE', ( #13875, #826, #2137, #7358 ) ) ;
#11168=DIRECTION ( 'NONE',  ( 1.000000000000000000, 0.000000000000000000, -0.000000000000000000 ) ) ;
#11180=DIRECTION ( 'NONE',  ( -0.2873478855663315623, -0.9578262852211555378, 1.261617073437858516E-13 ) ) ;
#11196=SURFACE_STYLE_USAGE ( .BOTH. , #8906 ) ;
#11213=CARTESIAN_POINT ( 'NONE',  ( 726.1975094929949819, 167.5243180396262801, -149.9999999999986358 ) ) ;
#11249=FACE_OUTER_BOUND ( 'NONE', #10582, .T. ) ;
#11251=ORIENTED_EDGE ( 'NONE', *, *, #6020, .T. ) ;
#11269=ORIENTED_EDGE ( 'NONE', *, *, #683, .F. ) ;
#11297=PLANE ( 'NONE',  #944 ) ;
#11300=CARTESIAN_POINT ( 'NONE',  ( 229.2257385731838042, 308.4724102386206255, 177.5999999999999091 ) ) ;
#11309=FACE_OUTER_BOUND ( 'NONE', #8299, .T. ) ;
#11328=VERTEX_POINT ( 'NONE', #10574 ) ;
#11335=VECTOR ( 'NONE', #7126, 1000.000000000000000 ) ;
#11368=ORIENTED_EDGE ( 'NONE', *, *, #12974, .T. ) ;
#11376=CARTESIAN_POINT ( 'NONE',  ( 716.7018481736364492, 193.3416907550361543, -182.8000000000001535 ) ) ;
#11379=ORIENTED_EDGE ( 'NONE', *, *, #1582, .T. ) ;
#11391=ORIENTED_EDGE ( 'NONE', *, *, #3489, .F. ) ;
#11392=ORIENTED_EDGE ( 'NONE', *, *, #12887, .T. ) ;
#11397=CARTESIAN_POINT ( 'NONE',  ( 707.5067158355135462, 162.6912496279608717, 177.6000000000001648 ) ) ;
#11431=VERTEX_POINT ( 'NONE', #597 ) ;
#11444=DIRECTION ( 'NONE',  ( -0.2873478855663477161, -0.9578262852211506528, 0.000000000000000000 ) ) ;
#11451=CARTESIAN_POINT ( 'NONE',  ( 708.1388811837595085, 164.7984674554473941, 177.6000000000000512 ) ) ;
#11465=ORIENTED_EDGE ( 'NONE', *, *, #13879, .F. ) ;
#11475=PRESENTATION_STYLE_ASSIGNMENT (( #11196 ) ) ;
#11495=FACE_OUTER_BOUND ( 'NONE', #2724, .T. ) ;
#11516=CARTESIAN_POINT ( 'NONE',  ( 227.7315295682384999, 303.4917135554678680, -177.6000000000004775 ) ) ;
#11520=ORIENTED_EDGE ( 'NONE', *, *, #7670, .F. ) ;
#11540=ORIENTED_EDGE ( 'NONE', *, *, #2963, .T. ) ;
#11544=EDGE_CURVE ( 'NONE', #10481, #12598, #3620, .T. ) ;
#11546=ADVANCED_FACE ( 'NONE', ( #3687 ), #2490, .T. ) ;
#11569=ORIENTED_EDGE ( 'NONE', *, *, #6020, .F. ) ;
#11621=ADVANCED_FACE ( 'NONE', ( #2872 ), #567, .F. ) ;
#11641=PLANE ( 'NONE',  #3793 ) ;
#11675=EDGE_CURVE ( 'NONE', #9054, #11431, #8551, .T. ) ;
#11699=CARTESIAN_POINT ( 'NONE',  ( 705.2654023280961155, 165.6605111121450591, -177.6000000000005627 ) ) ;
#11704=AXIS2_PLACEMENT_3D ( 'NONE', #11300, #10122, #11444 ) ;
#11718=ADVANCED_FACE ( 'NONE', ( #14521 ), #13337, .T. ) ;
#11721=EDGE_CURVE ( 'NONE', #10481, #4991, #8775, .T. ) ;
#11725=DIRECTION ( 'NONE',  ( -1.000000000000000000, -2.523234146875633539E-14, 0.000000000000000000 ) ) ;
#11741=CARTESIAN_POINT ( 'NONE',  ( 706.6446721788148579, 159.8177707722968819, -177.6000000000004775 ) ) ;
#11748=ORIENTED_EDGE ( 'NONE', *, *, #7670, .T. ) ;
#11752=EDGE_LOOP ( 'NONE', ( #196, #2031, #8815, #702 ) ) ;
#11761=CARTESIAN_POINT ( 'NONE',  ( 112.3905262037967105, 374.6350873459881541, -182.8000000000008640 ) ) ;
#11767=LINE ( 'NONE', #1744, #10353 ) ;
#11773=AXIS2_PLACEMENT_3D ( 'NONE', #10959, #834, #5352 ) ;
#11791=ORIENTED_EDGE ( 'NONE', *, *, #5732, .F. ) ;
#11796=DIRECTION ( 'NONE',  ( -0.2873478855663497700, -0.9578262852211499867, 0.000000000000000000 ) ) ;
#11800=COLOUR_RGB ( '',0.8941176470588234615, 0.8941176470588234615, 0.8941176470588234615 ) ;
#11806=VECTOR ( 'NONE', #4879, 1000.000000000000114 ) ;
#11815=LINE ( 'NONE', #1844, #7794 ) ;
#11817=ORIENTED_EDGE ( 'NONE', *, *, #12950, .T. ) ;
#11820=CARTESIAN_POINT ( 'NONE',  ( 708.1388811837593948, 164.7984674554467404, 177.6000000000001648 ) ) ;
#11836=VERTEX_POINT ( 'NONE', #7732 ) ;
#11841=DIRECTION ( 'NONE',  ( 0.2873478855663418874, 0.9578262852211524292, 0.000000000000000000 ) ) ;
#11878=DIRECTION ( 'NONE',  ( -0.000000000000000000, -0.000000000000000000, -1.000000000000000000 ) ) ;
#11884=CARTESIAN_POINT ( 'NONE',  ( 701.6639754956653405, 161.3119797772417883, 177.6000000000001648 ) ) ;
#11912=FACE_OUTER_BOUND ( 'NONE', #7818, .T. ) ;
#11917=EDGE_CURVE ( 'NONE', #12598, #1859, #2253, .T. ) ;
#11919=CARTESIAN_POINT ( 'NONE',  ( 228.5935732249376997, 306.3651924111334779, 182.7999999999996135 ) ) ;
#11930=VECTOR ( 'NONE', #109, 1000.000000000000000 ) ;
#11941=ORIENTED_EDGE ( 'NONE', *, *, #12887, .F. ) ;
#11964=DIRECTION ( 'NONE',  ( 0.9578262852211513190, -0.2873478855663454956, 0.000000000000000000 ) ) ;
#11979=EDGE_CURVE ( 'NONE', #5936, #2950, #8381, .T. ) ;
#11984=FACE_OUTER_BOUND ( 'NONE', #4653, .T. ) ;
#11994=DIRECTION ( 'NONE',  ( 0.2873478855663454401, 0.9578262852211514300, -3.927332483172771155E-15 ) ) ;
#12001=ORIENTED_EDGE ( 'NONE', *, *, #4356, .T. ) ;
#12002=CARTESIAN_POINT ( 'NONE',  ( 228.5935732249376997, 306.3651924111334779, 179.7999999999995850 ) ) ;
#12014=AXIS2_PLACEMENT_3D ( 'NONE', #2311, #10291, #5858 ) ;
#12037=EDGE_CURVE ( 'NONE', #2553, #6810, #9643, .T. ) ;
#12045=FACE_OUTER_BOUND ( 'NONE', #13245, .T. ) ;
#12047=VECTOR ( 'NONE', #3164, 1000.000000000000227 ) ;
#12075=CARTESIAN_POINT ( 'NONE',  ( 102.3333502089745934, 341.1111673632486259, -1.398642936228627705E-12 ) ) ;
#12078=PRODUCT_DEFINITION_FORMATION_WITH_SPECIFIED_SOURCE ( 'ANY', '', #6049, .NOT_KNOWN. ) ;
#12087=DIRECTION ( 'NONE',  ( 1.063400795443704616E-15, -3.190202386331113848E-16, -1.000000000000000000 ) ) ;
#12115=DIRECTION ( 'NONE',  ( -1.000000000000000000, 0.000000000000000000, 0.000000000000000000 ) ) ;
#12120=CARTESIAN_POINT ( 'NONE',  ( 708.1388811837590538, 164.7984674554467404, 177.5999999999999091 ) ) ;
#12145=EDGE_CURVE ( 'NONE', #2108, #10293, #5497, .T. ) ;
#12186=ORIENTED_EDGE ( 'NONE', *, *, #6557, .F. ) ;
#12197=DIRECTION ( 'NONE',  ( 1.063400795443704616E-15, -3.190202386331113848E-16, -1.000000000000000000 ) ) ;
#12221=VECTOR ( 'NONE', #10775, 1000.000000000000114 ) ;
#12306=DIRECTION ( 'NONE',  ( -0.9578262852211513190, 0.2873478855663453846, 0.000000000000000000 ) ) ;
#12310=LINE ( 'NONE', #2200, #3820 ) ;
#12373=VERTEX_POINT ( 'NONE', #9332 ) ;
#12378=CARTESIAN_POINT ( 'NONE',  ( 707.0389973793284071, 162.8315651648150606, -177.6000000000005059 ) ) ;
#12383=ADVANCED_FACE ( 'NONE', ( #13830 ), #2620, .F. ) ;
#12453=VECTOR ( 'NONE', #4540, 1000.000000000000227 ) ;
#12454=VECTOR ( 'NONE', #10108, 1000.000000000000000 ) ;
#12464=FACE_OUTER_BOUND ( 'NONE', #8277, .T. ) ;
#12465=AXIS2_PLACEMENT_3D ( 'NONE', #5374, #4131, #7512 ) ;
#12473=( GEOMETRIC_REPRESENTATION_CONTEXT ( 3 ) GLOBAL_UNCERTAINTY_ASSIGNED_CONTEXT ( ( #9156 ) ) GLOBAL_UNIT_ASSIGNED_CONTEXT ( ( #8453, #618, #13110 ) ) REPRESENTATION_CONTEXT ( 'NONE', 'WORKASPACE' ) );
#12474=DIRECTION ( 'NONE',  ( 0.9578262852211525402, -0.2873478855663419429, -0.000000000000000000 ) ) ;
#12488=ADVANCED_FACE ( 'NONE', ( #5197 ), #14206, .T. ) ;
#12504=DIRECTION ( 'NONE',  ( -0.9578262852211506528, 0.2873478855663477161, -0.000000000000000000 ) ) ;
#12506=ORIENTED_EDGE ( 'NONE', *, *, #10703, .T. ) ;
#12521=DIRECTION ( 'NONE',  ( 0.2873478855663483267, 0.9578262852211504308, 0.000000000000000000 ) ) ;
#12525=FACE_OUTER_BOUND ( 'NONE', #7141, .T. ) ;
#12534=CARTESIAN_POINT ( 'NONE',  ( 726.1975094929946408, 167.5243180396263938, 150.0000000000013642 ) ) ;
#12563=CARTESIAN_POINT ( 'NONE',  ( 708.1388811837592812, 164.7984674554473372, 182.8000000000001535 ) ) ;
#12571=LINE ( 'NONE', #10651, #188 ) ;
#12578=DIRECTION ( 'NONE',  ( 3.072361293536515954E-16, -4.159212477520619976E-15, -1.000000000000000000 ) ) ;
#12588=LINE ( 'NONE', #12734, #4052 ) ;
#12598=VERTEX_POINT ( 'NONE', #12563 ) ;
#12610=DIRECTION ( 'NONE',  ( 9.463134714538378657E-16, -7.093113185993356941E-16, -1.000000000000000000 ) ) ;
#12673=VERTEX_POINT ( 'NONE', #14488 ) ;
#12729=CARTESIAN_POINT ( 'NONE',  ( 707.0389973793288618, 162.8315651648156575, -177.6000000000005059 ) ) ;
#12734=CARTESIAN_POINT ( 'NONE',  ( 704.6332369798501531, 163.5532932846598726, 177.6000000000001648 ) ) ;
#12752=CARTESIAN_POINT ( 'NONE',  ( 601.4378431141739156, -180.4313529342555000, 9.352357694252897163E-13 ) ) ;
#12771=DIRECTION ( 'NONE',  ( -0.9578262852211514300, 0.2873478855663452736, -1.110223024625156540E-15 ) ) ;
#12828=CARTESIAN_POINT ( 'NONE',  ( 227.7315295682384999, 303.4917135554678680, -177.6000000000009038 ) ) ;
#12839=ORIENTED_EDGE ( 'NONE', *, *, #1457, .F. ) ;
#12841=VERTEX_POINT ( 'NONE', #14105 ) ;
#12842=VERTEX_POINT ( 'NONE', #8494 ) ;
#12857=ORIENTED_EDGE ( 'NONE', *, *, #698, .F. ) ;
#12880=FACE_OUTER_BOUND ( 'NONE', #11752, .T. ) ;
#12887=EDGE_CURVE ( 'NONE', #5667, #11071, #8792, .T. ) ;
#12919=CARTESIAN_POINT ( 'NONE',  ( 125.3981793592653702, -37.61945380778043102, -182.7999999999979934 ) ) ;
#12928=CARTESIAN_POINT ( 'NONE',  ( 702.5260191523636877, 164.1854586329052097, 150.0000000000013358 ) ) ;
#12944=AXIS2_PLACEMENT_3D ( 'NONE', #12752, #10686, #13053 ) ;
#12950=EDGE_CURVE ( 'NONE', #12598, #10624, #4225, .T. ) ;
#12969=VECTOR ( 'NONE', #11120, 1000.000000000000000 ) ;
#12974=EDGE_CURVE ( 'NONE', #6810, #10436, #10032, .T. ) ;
#12988=ORIENTED_EDGE ( 'NONE', *, *, #13526, .T. ) ;
#13053=DIRECTION ( 'NONE',  ( -0.2873478855663502141, -0.9578262852211498757, 0.000000000000000000 ) ) ;
#13058=ADVANCED_FACE ( 'NONE', ( #10189 ), #2206, .F. ) ;
#13069=EDGE_CURVE ( 'NONE', #5667, #9054, #3245, .T. ) ;
#13071=LINE ( 'NONE', #10850, #9924 ) ;
#13076=DIRECTION ( 'NONE',  ( 0.9578262852211507639, -0.2873478855663477716, 0.000000000000000000 ) ) ;
#13110=( NAMED_UNIT ( * ) SI_UNIT ( $, .STERADIAN. ) SOLID_ANGLE_UNIT ( ) );
#13153=ORIENTED_EDGE ( 'NONE', *, *, #1577, .F. ) ;
#13164=DIRECTION ( 'NONE',  ( 0.2873478855663315068, 0.9578262852211555378, 0.000000000000000000 ) ) ;
#13168=VECTOR ( 'NONE', #6848, 1000.000000000000227 ) ;
#13174=CARTESIAN_POINT ( 'NONE',  ( 716.7018481736364492, 193.3416907550361543, -182.8000000000001819 ) ) ;
#13186=ORIENTED_EDGE ( 'NONE', *, *, #13694, .T. ) ;
#13201=EDGE_CURVE ( 'NONE', #13316, #11071, #8698, .T. ) ;
#13205=VECTOR ( 'NONE', #1239, 1000.000000000000000 ) ;
#13215=ORIENTED_EDGE ( 'NONE', *, *, #11675, .T. ) ;
#13237=FACE_OUTER_BOUND ( 'NONE', #3275, .T. ) ;
#13242=ORIENTED_EDGE ( 'NONE', *, *, #647, .T. ) ;
#13245=EDGE_LOOP ( 'NONE', ( #10397, #3844, #831, #14261 ) ) ;
#13252=LINE ( 'NONE', #6464, #10632 ) ;
#13253=ORIENTED_EDGE ( 'NONE', *, *, #6129, .T. ) ;
#13254=ORIENTED_EDGE ( 'NONE', *, *, #8085, .T. ) ;
#13259=DIRECTION ( 'NONE',  ( -0.9578262852211498757, 0.2873478855663503251, -1.198990317802636355E-15 ) ) ;
#13264=VECTOR ( 'NONE', #334, 1000.000000000000000 ) ;
#13285=LINE ( 'NONE', #2957, #3474 ) ;
#13292=ORIENTED_EDGE ( 'NONE', *, *, #7111, .T. ) ;
#13316=VERTEX_POINT ( 'NONE', #10721 ) ;
#13337=PLANE ( 'NONE',  #13975 ) ;
#13341=ORIENTED_EDGE ( 'NONE', *, *, #5914, .F. ) ;
#13349=LINE ( 'NONE', #14316, #7239 ) ;
#13367=DIRECTION ( 'NONE',  ( -1.148424442117026787E-15, 3.445273326351093279E-16, 1.000000000000000000 ) ) ;
#13397=LINE ( 'NONE', #7659, #7574 ) ;
#13400=CARTESIAN_POINT ( 'NONE',  ( 723.8855453127956707, 217.2873478855657368, -6.736265118569116382E-13 ) ) ;
#13415=AXIS2_PLACEMENT_3D ( 'NONE', #6404, #4178, #3075 ) ;
#13470=CIRCLE ( 'NONE', #7817, 2.199999999999746159 ) ;
#13492=( NAMED_UNIT ( * ) PLANE_ANGLE_UNIT ( ) SI_UNIT ( $, .RADIAN. ) );
#13493=AXIS2_PLACEMENT_3D ( 'NONE', #2430, #1316, #5890 ) ;
#13495=CARTESIAN_POINT ( 'NONE',  ( 705.2654023280961155, 165.6605111121464518, 177.6000000000000512 ) ) ;
#13496=ORIENTED_EDGE ( 'NONE', *, *, #14584, .F. ) ;
#13501=VECTOR ( 'NONE', #554, 1000.000000000000227 ) ;
#13526=EDGE_CURVE ( 'NONE', #2452, #12673, #10833, .T. ) ;
#13528=FACE_OUTER_BOUND ( 'NONE', #3733, .T. ) ;
#13532=ORIENTED_EDGE ( 'NONE', *, *, #547, .F. ) ;
#13555=CARTESIAN_POINT ( 'NONE',  ( 708.1388811837592812, 164.7984674554467404, -177.6000000000002217 ) ) ;
#13558=ORIENTED_EDGE ( 'NONE', *, *, #1515, .F. ) ;
#13563=CARTESIAN_POINT ( 'NONE',  ( 708.1388811837593948, 164.7984674554474225, 177.6000000000001648 ) ) ;
#13580=ORIENTED_EDGE ( 'NONE', *, *, #1582, .F. ) ;
#13585=ADVANCED_FACE ( 'NONE', ( #5581 ), #6628, .F. ) ;
#13593=CARTESIAN_POINT ( 'NONE',  ( 708.1388811837596222, 164.7984674554460014, -177.6000000000005343 ) ) ;
#13596=CARTESIAN_POINT ( 'NONE',  ( 703.1581845006096501, 166.2926764603917036, 177.6000000000001648 ) ) ;
#13600=CIRCLE ( 'NONE', #13636, 2.199999999999757705 ) ;
#13623=DIRECTION ( 'NONE',  ( -0.9578262852211525402, 0.2873478855663419429, 0.000000000000000000 ) ) ;
#13636=AXIS2_PLACEMENT_3D ( 'NONE', #8190, #13972, #11725 ) ;
#13644=EDGE_LOOP ( 'NONE', ( #3097, #6492, #4338, #13834 ) ) ;
#13666=CARTESIAN_POINT ( 'NONE',  ( 237.7887055630606028, 337.0156335382089310, -182.8000000000007219 ) ) ;
#13686=FACE_OUTER_BOUND ( 'NONE', #11161, .T. ) ;
#13694=EDGE_CURVE ( 'NONE', #5236, #11071, #11126, .T. ) ;
#13701=( GEOMETRIC_REPRESENTATION_CONTEXT ( 3 ) GLOBAL_UNCERTAINTY_ASSIGNED_CONTEXT ( ( #3704 ) ) GLOBAL_UNIT_ASSIGNED_CONTEXT ( ( #3524, #1370, #5801 ) ) REPRESENTATION_CONTEXT ( 'NONE', 'WORKASPACE' ) );
#13712=CARTESIAN_POINT ( 'NONE',  ( 604.3113219698370813, -181.2933965909541598, 182.8000000000001535 ) ) ;
#13722=LINE ( 'NONE', #12828, #7809 ) ;
#13723=EDGE_CURVE ( 'NONE', #14148, #14518, #10593, .T. ) ;
#13727=ADVANCED_FACE ( 'NONE', ( #166 ), #14070, .F. ) ;
#13729=CARTESIAN_POINT ( 'NONE',  ( 708.1388811837593948, 164.7984674554466551, -182.7999999999999545 ) ) ;
#13748=DIRECTION ( 'NONE',  ( 0.2873478855663417764, 0.9578262852211525402, 0.000000000000000000 ) ) ;
#13780=PLANE ( 'NONE',  #7304 ) ;
#13795=ADVANCED_FACE ( 'NONE', ( #9570 ), #13780, .F. ) ;
#13808=CARTESIAN_POINT ( 'NONE',  ( 229.2257385731836621, 308.4724102386199434, 182.7999999999996135 ) ) ;
#13813=DIRECTION ( 'NONE',  ( 0.9578262852211525402, -0.2873478855663417764, 1.110223024625127747E-15 ) ) ;
#13830=FACE_OUTER_BOUND ( 'NONE', #7839, .T. ) ;
#13834=ORIENTED_EDGE ( 'NONE', *, *, #880, .T. ) ;
#13835=LINE ( 'NONE', #12729, #11335 ) ;
#13847=ORIENTED_EDGE ( 'NONE', *, *, #683, .T. ) ;
#13853=ORIENTED_EDGE ( 'NONE', *, *, #8635, .T. ) ;
#13875=ORIENTED_EDGE ( 'NONE', *, *, #7406, .T. ) ;
#13878=LINE ( 'NONE', #13808, #4738 ) ;
#13879=EDGE_CURVE ( 'NONE', #8002, #2622, #14144, .T. ) ;
#13908=AXIS2_PLACEMENT_3D ( 'NONE', #4924, #3669, #3826 ) ;
#13918=DIRECTION ( 'NONE',  ( -0.9578262852211525402, 0.2873478855663419429, 0.000000000000000000 ) ) ;
#13925=CARTESIAN_POINT ( 'NONE',  ( 237.7887055630606312, 337.0156335382089310, -182.8000000000007219 ) ) ;
#13931=VECTOR ( 'NONE', #5839, 1000.000000000000000 ) ;
#13936=ADVANCED_FACE ( 'NONE', ( #11984 ), #10895, .F. ) ;
#13947=DIRECTION ( 'NONE',  ( 0.2873478855663503806, 0.9578262852211499867, -3.544669318145085478E-17 ) ) ;
#13969=DIRECTION ( 'NONE',  ( 0.2873478855663417764, 0.9578262852211525402, -6.938893903907204712E-15 ) ) ;
#13972=DIRECTION ( 'NONE',  ( 0.000000000000000000, 0.000000000000000000, 1.000000000000000000 ) ) ;
#13975=AXIS2_PLACEMENT_3D ( 'NONE', #10017, #14457, #4272 ) ;
#13976=LINE ( 'NONE', #9470, #13931 ) ;
#14006=ORIENTED_EDGE ( 'NONE', *, *, #1525, .F. ) ;
#14015=CARTESIAN_POINT ( 'NONE',  ( 703.1581845006096501, 166.2926764603917036, 177.6000000000001648 ) ) ;
#14034=PRODUCT_DEFINITION_CONTEXT ( 'detailed design', #3296, 'design' ) ;
#14068=EDGE_LOOP ( 'NONE', ( #13341, #13153, #9243, #10209 ) ) ;
#14070=CYLINDRICAL_SURFACE ( 'NONE', #13908, 2.199999999999702194 ) ;
#14084=VECTOR ( 'NONE', #1558, 1000.000000000000000 ) ;
#14094=CIRCLE ( 'NONE', #167, 5.199999999999760369 ) ;
#14105=CARTESIAN_POINT ( 'NONE',  ( 237.7887055630607733, 337.0156335382104089, 179.7999999999995850 ) ) ;
#14144=LINE ( 'NONE', #9931, #14611 ) ;
#14148=VERTEX_POINT ( 'NONE', #11741 ) ;
#14150=ADVANCED_FACE ( 'NONE', ( #13686 ), #10358, .T. ) ;
#14158=VECTOR ( 'NONE', #7162, 1000.000000000000114 ) ;
#14206=PLANE ( 'NONE',  #7974 ) ;
#14234=CARTESIAN_POINT ( 'NONE',  ( 703.1581845006096501, 166.2926764603917036, -149.9999999999986642 ) ) ;
#14239=DIRECTION ( 'NONE',  ( 0.000000000000000000, 0.000000000000000000, 1.000000000000000000 ) ) ;
#14260=ORIENTED_EDGE ( 'NONE', *, *, #764, .T. ) ;
#14261=ORIENTED_EDGE ( 'NONE', *, *, #9307, .T. ) ;
#14271=CARTESIAN_POINT ( 'NONE',  ( 229.2257385731836905, 308.4724102386184654, -179.8000000000005230 ) ) ;
#14281=EDGE_CURVE ( 'NONE', #5236, #11328, #6445, .T. ) ;
#14302=DIRECTION ( 'NONE',  ( 0.000000000000000000, 0.000000000000000000, 1.000000000000000000 ) ) ;
#14303=VERTEX_POINT ( 'NONE', #10727 ) ;
#14305=LINE ( 'NONE', #795, #6070 ) ;
#14313=VECTOR ( 'NONE', #10514, 1000.000000000000000 ) ;
#14316=CARTESIAN_POINT ( 'NONE',  ( 723.8855453127953297, 217.2873478855664757, 177.5999999999999659 ) ) ;
#14318=ORIENTED_EDGE ( 'NONE', *, *, #1821, .T. ) ;
#14319=ADVANCED_FACE ( 'NONE', ( #7827 ), #5060, .F. ) ;
#14359=VECTOR ( 'NONE', #14473, 1000.000000000000114 ) ;
#14364=ORIENTED_EDGE ( 'NONE', *, *, #9307, .F. ) ;
#14366=AXIS2_PLACEMENT_3D ( 'NONE', #7814, #12087, #9955 ) ;
#14375=VECTOR ( 'NONE', #4275, 1000.000000000000114 ) ;
#14380=CARTESIAN_POINT ( 'NONE',  ( 723.3240306373314752, 157.9460551874147427, -149.9999999999986358 ) ) ;
#14419=CARTESIAN_POINT ( 'NONE',  ( 604.3113219698374223, -181.2933965909545293, 9.397040286797935582E-13 ) ) ;
#14457=DIRECTION ( 'NONE',  ( 0.9578262852211525402, -0.2873478855663419429, -0.000000000000000000 ) ) ;
#14473=DIRECTION ( 'NONE',  ( -0.2873478855663418874, -0.9578262852211524292, -1.261617073437818631E-13 ) ) ;
#14488=CARTESIAN_POINT ( 'NONE',  ( 702.5260191523638014, 164.1854586329053518, 177.6000000000001648 ) ) ;
#14515=PRODUCT_DEFINITION ( 'UNKNOWN', '', #12078, #14034 ) ;
#14516=CARTESIAN_POINT ( 'NONE',  ( 708.1388811837593948, 164.7984674554458593, -182.7999999999999261 ) ) ;
#14518=VERTEX_POINT ( 'NONE', #13729 ) ;
#14521=FACE_OUTER_BOUND ( 'NONE', #14068, .T. ) ;
#14558=ORIENTED_EDGE ( 'NONE', *, *, #3217, .F. ) ;
#14584=EDGE_CURVE ( 'NONE', #4991, #12841, #9663, .T. ) ;
#14591=CARTESIAN_POINT ( 'NONE',  ( 707.5067158355136598, 162.6912496279593938, -177.6000000000005059 ) ) ;
#14592=ADVANCED_FACE ( 'NONE', ( #2569 ), #11641, .F. ) ;
#14596=SURFACE_STYLE_FILL_AREA ( #10088 ) ;
#14611=VECTOR ( 'NONE', #8444, 1000.000000000000000 ) ;
#14682=COLOUR_RGB('Off White',0.89,0.88,0.83);
#14683=FILL_AREA_STYLE_COLOUR('',#14682);
#14684=FILL_AREA_STYLE('',(#14683));
#14685=SURFACE_STYLE_FILL_AREA(#14684);
#14686=SURFACE_SIDE_STYLE('',(#14685));
#14687=SURFACE_STYLE_USAGE(.BOTH.,#14686);
#14688=PRESENTATION_STYLE_ASSIGNMENT((#14687));
ENDSEC;
END-ISO-10303-21;
